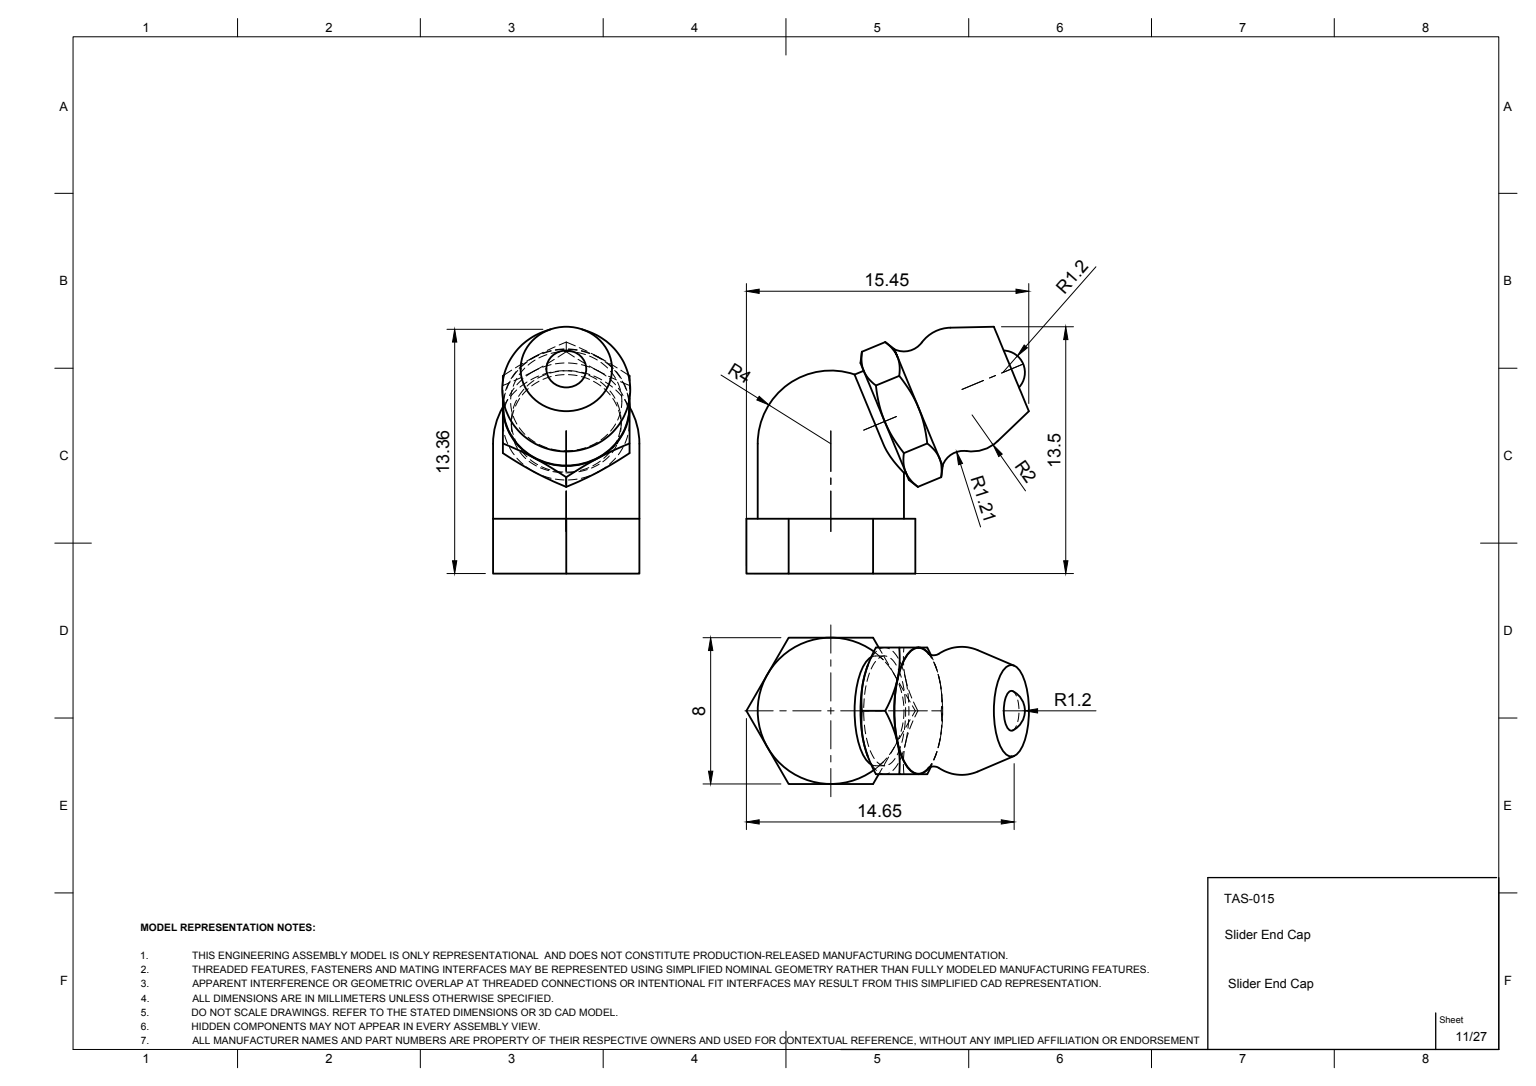
ISO-10303-21;
HEADER;
/* Generated by software containing ST-Developer
 * from STEP Tools, Inc. (www.steptools.com) 
 */

FILE_DESCRIPTION(
/* description */ ('STEP AP214'),
/* implementation_level */ '2;1');

FILE_NAME(
/* name */ 'Slider End Cap.step',
/* time_stamp */ '2026-11-15T14:49:54-08:00',
/* author */ (''),
/* organization */ (''),
/* preprocessor_version */ 'ST-DEVELOPER v20.2',
/* originating_system */ 'Autodesk Translation Framework v15.17.0.0',
/* authorisation */ '');

FILE_SCHEMA (('AUTOMOTIVE_DESIGN { 1 0 10303 214 3 1 1 }'));
ENDSEC;

DATA;
#10=MECHANICAL_DESIGN_GEOMETRIC_PRESENTATION_REPRESENTATION('',(#1106),#66721);
#35=SPHERICAL_SURFACE('',#27201,1.2);
#36=SPHERICAL_SURFACE('',#27220,4.);
#69=TOROIDAL_SURFACE('',#27193,4.25,1.21);
#83=(
BOUNDED_CURVE()
B_SPLINE_CURVE(2,(#39567,#39568,#39569),.UNSPECIFIED.,.F.,.F.)
B_SPLINE_CURVE_WITH_KNOTS((3,3),(-1.38994780338837,-1.00314154055664),
 .UNSPECIFIED.)
CURVE()
GEOMETRIC_REPRESENTATION_ITEM()
RATIONAL_B_SPLINE_CURVE((1.79495951130746,1.93380011269289,1.93380011269289))
REPRESENTATION_ITEM('')
);
#84=(
BOUNDED_CURVE()
B_SPLINE_CURVE(2,(#39570,#39571,#39572),.UNSPECIFIED.,.F.,.F.)
B_SPLINE_CURVE_WITH_KNOTS((3,3),(-1.00619430729118,-0.618602381117838),
 .UNSPECIFIED.)
CURVE()
GEOMETRIC_REPRESENTATION_ITEM()
RATIONAL_B_SPLINE_CURVE((1.93745653739061,1.93745653739061,1.7983534165231))
REPRESENTATION_ITEM('')
);
#85=(
BOUNDED_CURVE()
B_SPLINE_CURVE(2,(#39578,#39579,#39580),.UNSPECIFIED.,.F.,.F.)
B_SPLINE_CURVE_WITH_KNOTS((3,3),(-1.38994780338837,-1.00314154055664),
 .UNSPECIFIED.)
CURVE()
GEOMETRIC_REPRESENTATION_ITEM()
RATIONAL_B_SPLINE_CURVE((1.79495951130745,1.93380011269288,1.93380011269288))
REPRESENTATION_ITEM('')
);
#86=(
BOUNDED_CURVE()
B_SPLINE_CURVE(2,(#39581,#39582,#39583),.UNSPECIFIED.,.F.,.F.)
B_SPLINE_CURVE_WITH_KNOTS((3,3),(-1.00619430729117,-0.618602381117832),
 .UNSPECIFIED.)
CURVE()
GEOMETRIC_REPRESENTATION_ITEM()
RATIONAL_B_SPLINE_CURVE((1.9374565373906,1.9374565373906,1.79835341652309))
REPRESENTATION_ITEM('')
);
#87=(
BOUNDED_CURVE()
B_SPLINE_CURVE(2,(#39705,#39706,#39707),.UNSPECIFIED.,.F.,.F.)
B_SPLINE_CURVE_WITH_KNOTS((3,3),(-1.14357963809553,-0.720457873954785),
 .UNSPECIFIED.)
CURVE()
GEOMETRIC_REPRESENTATION_ITEM()
RATIONAL_B_SPLINE_CURVE((2.10284386262275,2.10284386262275,1.95186646604709))
REPRESENTATION_ITEM('')
);
#88=(
BOUNDED_CURVE()
B_SPLINE_CURVE(2,(#39708,#39709,#39710),.UNSPECIFIED.,.F.,.F.)
B_SPLINE_CURVE_WITH_KNOTS((3,3),(-1.51402948258723,-1.10175646251728),
 .UNSPECIFIED.)
CURVE()
GEOMETRIC_REPRESENTATION_ITEM()
RATIONAL_B_SPLINE_CURVE((1.90498640166842,2.0523376126434,2.0523376126434))
REPRESENTATION_ITEM('')
);
#89=(
BOUNDED_CURVE()
B_SPLINE_CURVE(2,(#39713,#39714,#39715),.UNSPECIFIED.,.F.,.F.)
B_SPLINE_CURVE_WITH_KNOTS((3,3),(-1.00619430729147,-0.618602381118052),
 .UNSPECIFIED.)
CURVE()
GEOMETRIC_REPRESENTATION_ITEM()
RATIONAL_B_SPLINE_CURVE((1.93745653739095,1.93745653739095,1.79835341652342))
REPRESENTATION_ITEM('')
);
#90=(
BOUNDED_CURVE()
B_SPLINE_CURVE(2,(#39716,#39717,#39718),.UNSPECIFIED.,.F.,.F.)
B_SPLINE_CURVE_WITH_KNOTS((3,3),(-1.59428966155348,-1.16547770853232),
 .UNSPECIFIED.)
CURVE()
GEOMETRIC_REPRESENTATION_ITEM()
RATIONAL_B_SPLINE_CURVE((1.97645710138757,2.12933659022722,2.12933659022723))
REPRESENTATION_ITEM('')
);
#91=(
BOUNDED_CURVE()
B_SPLINE_CURVE(2,(#39721,#39722,#39723),.UNSPECIFIED.,.F.,.F.)
B_SPLINE_CURVE_WITH_KNOTS((3,3),(-1.39378623346489,-1.00619430729147),
 .UNSPECIFIED.)
CURVE()
GEOMETRIC_REPRESENTATION_ITEM()
RATIONAL_B_SPLINE_CURVE((1.79835341652342,1.93745653739095,1.93745653739095))
REPRESENTATION_ITEM('')
);
#92=(
BOUNDED_CURVE()
B_SPLINE_CURVE(2,(#39724,#39725,#39726),.UNSPECIFIED.,.F.,.F.)
B_SPLINE_CURVE_WITH_KNOTS((3,3),(-1.00314154055692,-0.616335277725119),
 .UNSPECIFIED.)
CURVE()
GEOMETRIC_REPRESENTATION_ITEM()
RATIONAL_B_SPLINE_CURVE((1.93380011269323,1.93380011269323,1.79495951130777))
REPRESENTATION_ITEM('')
);
#93=(
BOUNDED_CURVE()
B_SPLINE_CURVE(2,(#39729,#39730,#39731),.UNSPECIFIED.,.F.,.F.)
B_SPLINE_CURVE_WITH_KNOTS((3,3),(-1.38994780338873,-1.00314154055692),
 .UNSPECIFIED.)
CURVE()
GEOMETRIC_REPRESENTATION_ITEM()
RATIONAL_B_SPLINE_CURVE((1.79495951130777,1.93380011269323,1.93380011269323))
REPRESENTATION_ITEM('')
);
#94=(
BOUNDED_CURVE()
B_SPLINE_CURVE(2,(#39732,#39733,#39734),.UNSPECIFIED.,.F.,.F.)
B_SPLINE_CURVE_WITH_KNOTS((3,3),(-1.16547770853232,-0.73666575551116),
 .UNSPECIFIED.)
CURVE()
GEOMETRIC_REPRESENTATION_ITEM()
RATIONAL_B_SPLINE_CURVE((2.12933659022723,2.12933659022723,1.97645710138758))
REPRESENTATION_ITEM('')
);
#95=(
BOUNDED_CURVE()
B_SPLINE_CURVE(2,(#39737,#39738,#39739),.UNSPECIFIED.,.F.,.F.)
B_SPLINE_CURVE_WITH_KNOTS((3,3),(-1.56670140223628,-1.14357963809553),
 .UNSPECIFIED.)
CURVE()
GEOMETRIC_REPRESENTATION_ITEM()
RATIONAL_B_SPLINE_CURVE((1.95186646604709,2.10284386262275,2.10284386262275))
REPRESENTATION_ITEM('')
);
#96=(
BOUNDED_CURVE()
B_SPLINE_CURVE(2,(#39740,#39741,#39742),.UNSPECIFIED.,.F.,.F.)
B_SPLINE_CURVE_WITH_KNOTS((3,3),(-1.09872453323964,-0.687236958819027),
 .UNSPECIFIED.)
CURVE()
GEOMETRIC_REPRESENTATION_ITEM()
RATIONAL_B_SPLINE_CURVE((2.04868118794568,2.04868118794568,1.90159249645282))
REPRESENTATION_ITEM('')
);
#97=(
BOUNDED_CURVE()
B_SPLINE_CURVE(2,(#39745,#39746,#39747),.UNSPECIFIED.,.F.,.F.)
B_SPLINE_CURVE_WITH_KNOTS((3,3),(-1.56670140224009,-1.14357963809856),
 .UNSPECIFIED.)
CURVE()
GEOMETRIC_REPRESENTATION_ITEM()
RATIONAL_B_SPLINE_CURVE((1.9518664660505,2.10284386262641,2.10284386262641))
REPRESENTATION_ITEM('')
);
#98=(
BOUNDED_CURVE()
B_SPLINE_CURVE(2,(#39748,#39749,#39750),.UNSPECIFIED.,.F.,.F.)
B_SPLINE_CURVE_WITH_KNOTS((3,3),(-1.10777980342349,-0.69394596557458),
 .UNSPECIFIED.)
CURVE()
GEOMETRIC_REPRESENTATION_ITEM()
RATIONAL_B_SPLINE_CURVE((2.05960365436383,2.05960365436383,1.91173076506448))
REPRESENTATION_ITEM('')
);
#99=(
BOUNDED_CURVE()
B_SPLINE_CURVE(2,(#39753,#39754,#39755),.UNSPECIFIED.,.F.,.F.)
B_SPLINE_CURVE_WITH_KNOTS((3,3),(-1.40141169651805,-1.01225852375907),
 .UNSPECIFIED.)
CURVE()
GEOMETRIC_REPRESENTATION_ITEM()
RATIONAL_B_SPLINE_CURVE((1.80509777991977,1.94472257911162,1.94472257911162))
REPRESENTATION_ITEM('')
);
#100=(
BOUNDED_CURVE()
B_SPLINE_CURVE(2,(#39756,#39757,#39758),.UNSPECIFIED.,.F.,.F.)
B_SPLINE_CURVE_WITH_KNOTS((3,3),(-1.16547770853319,-0.736665755511809),
 .UNSPECIFIED.)
CURVE()
GEOMETRIC_REPRESENTATION_ITEM()
RATIONAL_B_SPLINE_CURVE((2.12933659022829,2.12933659022829,1.97645710138856))
REPRESENTATION_ITEM('')
);
#101=(
BOUNDED_CURVE()
B_SPLINE_CURVE(2,(#39761,#39762,#39763),.UNSPECIFIED.,.F.,.F.)
B_SPLINE_CURVE_WITH_KNOTS((3,3),(-1.40141169651807,-1.01225852375909),
 .UNSPECIFIED.)
CURVE()
GEOMETRIC_REPRESENTATION_ITEM()
RATIONAL_B_SPLINE_CURVE((1.80509777991979,1.94472257911164,1.94472257911164))
REPRESENTATION_ITEM('')
);
#102=(
BOUNDED_CURVE()
B_SPLINE_CURVE(2,(#39764,#39765,#39766),.UNSPECIFIED.,.F.,.F.)
B_SPLINE_CURVE_WITH_KNOTS((3,3),(-1.01225852375907,-0.623105351000092),
 .UNSPECIFIED.)
CURVE()
GEOMETRIC_REPRESENTATION_ITEM()
RATIONAL_B_SPLINE_CURVE((1.94472257911162,1.94472257911162,1.80509777991977))
REPRESENTATION_ITEM('')
);
#103=(
BOUNDED_CURVE()
B_SPLINE_CURVE(2,(#39769,#39770,#39771),.UNSPECIFIED.,.F.,.F.)
B_SPLINE_CURVE_WITH_KNOTS((3,3),(-1.59428966155458,-1.16547770853319),
 .UNSPECIFIED.)
CURVE()
GEOMETRIC_REPRESENTATION_ITEM()
RATIONAL_B_SPLINE_CURVE((1.97645710138856,2.12933659022828,2.12933659022828))
REPRESENTATION_ITEM('')
);
#104=(
BOUNDED_CURVE()
B_SPLINE_CURVE(2,(#39772,#39773,#39774),.UNSPECIFIED.,.F.,.F.)
B_SPLINE_CURVE_WITH_KNOTS((3,3),(-1.01225852375909,-0.623105351000104),
 .UNSPECIFIED.)
CURVE()
GEOMETRIC_REPRESENTATION_ITEM()
RATIONAL_B_SPLINE_CURVE((1.94472257911164,1.94472257911164,1.80509777991979))
REPRESENTATION_ITEM('')
);
#105=(
BOUNDED_CURVE()
B_SPLINE_CURVE(2,(#39777,#39778,#39779),.UNSPECIFIED.,.F.,.F.)
B_SPLINE_CURVE_WITH_KNOTS((3,3),(-1.52161364127241,-1.1077798034235),
 .UNSPECIFIED.)
CURVE()
GEOMETRIC_REPRESENTATION_ITEM()
RATIONAL_B_SPLINE_CURVE((1.91173076506449,2.05960365436384,2.05960365436384))
REPRESENTATION_ITEM('')
);
#106=(
BOUNDED_CURVE()
B_SPLINE_CURVE(2,(#39780,#39781,#39782),.UNSPECIFIED.,.F.,.F.)
B_SPLINE_CURVE_WITH_KNOTS((3,3),(-1.14357963809856,-0.720457873957025),
 .UNSPECIFIED.)
CURVE()
GEOMETRIC_REPRESENTATION_ITEM()
RATIONAL_B_SPLINE_CURVE((2.10284386262641,2.10284386262641,1.95186646605049))
REPRESENTATION_ITEM('')
);
#115=B_SPLINE_CURVE_WITH_KNOTS('',3,(#39589,#39590,#39591,#39592,#39593,
#39594,#39595,#39596,#39597,#39598),.UNSPECIFIED.,.F.,.F.,(4,2,2,2,4),(0.112312904835896,
0.113244103065848,0.226488206131697,0.343893756973101,0.461299307814506),
 .UNSPECIFIED.);
#116=B_SPLINE_CURVE_WITH_KNOTS('',3,(#39602,#39603,#39604,#39605,#39606,
#39607,#39608,#39609,#39610,#39611),.UNSPECIFIED.,.F.,.F.,(4,2,2,2,4),(0.461299307814506,
0.57870485865591,0.696110409497315,0.809354512563163,0.810285710793116),
 .UNSPECIFIED.);
#403=(
BOUNDED_SURFACE()
B_SPLINE_SURFACE(2,2,((#39525,#39526,#39527,#39528,#39529,#39530,#39531,
#39532,#39533),(#39534,#39535,#39536,#39537,#39538,#39539,#39540,#39541,
#39542),(#39543,#39544,#39545,#39546,#39547,#39548,#39549,#39550,#39551)),
 .UNSPECIFIED.,.F.,.T.,.F.)
B_SPLINE_SURFACE_WITH_KNOTS((3,3),(3,2,2,2,3),(-0.371257902576148,0.541962924803503),
(-3.14159265358979,-1.5707963267949,0.,1.5707963267949,3.14159265358979),
 .UNSPECIFIED.)
GEOMETRIC_REPRESENTATION_ITEM()
RATIONAL_B_SPLINE_SURFACE(((1.,0.707106781186548,1.,0.707106781186548,1.,
0.707106781186548,1.,0.707106781186548,1.),(0.897552147568833,0.634665210014471,
0.897552147568833,0.634665210014471,0.897552147568833,0.634665210014471,
0.897552147568833,0.634665210014471,0.897552147568833),(1.,0.707106781186548,
1.,0.707106781186548,1.,0.707106781186548,1.,0.707106781186548,1.)))
REPRESENTATION_ITEM('')
SURFACE()
);
#528=CONICAL_SURFACE('',#27199,2.5,0.371257902576146);
#529=CONICAL_SURFACE('',#27203,4.00000000000001,1.04719755119661);
#530=CONICAL_SURFACE('',#27205,3.46410161513776,1.0471975511966);
#531=CONICAL_SURFACE('',#27247,3.46410161513776,1.0471975511966);
#532=CONICAL_SURFACE('',#27248,3.46410161513776,1.0471975511966);
#533=CONICAL_SURFACE('',#27249,3.46410161513776,1.0471975511966);
#534=CONICAL_SURFACE('',#27250,3.46410161513776,1.0471975511966);
#535=CONICAL_SURFACE('',#27251,3.46410161513776,1.0471975511966);
#536=CONICAL_SURFACE('',#27252,4.00000000000001,1.04719755119661);
#537=CONICAL_SURFACE('',#27253,4.00000000000001,1.04719755119661);
#538=CONICAL_SURFACE('',#27254,4.00000000000001,1.04719755119661);
#539=CONICAL_SURFACE('',#27255,4.00000000000001,1.04719755119661);
#540=CONICAL_SURFACE('',#27256,4.00000000000001,1.04719755119661);
#1044=SHAPE_REPRESENTATION_RELATIONSHIP('SRR','None',#66902,#1075);
#1075=ADVANCED_BREP_SHAPE_REPRESENTATION('',(#1141),#66693);
#1106=STYLED_ITEM('',(#67095),#1141);
#1141=MANIFOLD_SOLID_BREP('Body1',#25672);
#1299=FACE_BOUND('',#4423,.T.);
#1300=FACE_BOUND('',#4425,.T.);
#1301=FACE_BOUND('',#4456,.T.);
#1848=PLANE('',#27222);
#1849=PLANE('',#27228);
#1850=PLANE('',#27234);
#1851=PLANE('',#27235);
#1852=PLANE('',#27236);
#1853=PLANE('',#27237);
#1854=PLANE('',#27238);
#1855=PLANE('',#27239);
#1856=PLANE('',#27240);
#1857=PLANE('',#27241);
#1858=PLANE('',#27242);
#1859=PLANE('',#27243);
#1860=PLANE('',#27244);
#1861=PLANE('',#27245);
#1862=PLANE('',#27246);
#1863=PLANE('',#27257);
#1864=PLANE('',#27258);
#1865=PLANE('',#27259);
#1866=PLANE('',#27260);
#1867=PLANE('',#27261);
#1868=PLANE('',#27262);
#1869=PLANE('',#27263);
#2840=FACE_OUTER_BOUND('',#4413,.T.);
#2841=FACE_OUTER_BOUND('',#4414,.T.);
#2842=FACE_OUTER_BOUND('',#4415,.T.);
#2843=FACE_OUTER_BOUND('',#4416,.T.);
#2844=FACE_OUTER_BOUND('',#4417,.T.);
#2845=FACE_OUTER_BOUND('',#4418,.T.);
#2846=FACE_OUTER_BOUND('',#4419,.T.);
#2847=FACE_OUTER_BOUND('',#4420,.T.);
#2848=FACE_OUTER_BOUND('',#4421,.T.);
#2849=FACE_OUTER_BOUND('',#4422,.T.);
#2850=FACE_OUTER_BOUND('',#4424,.T.);
#2851=FACE_OUTER_BOUND('',#4426,.T.);
#2852=FACE_OUTER_BOUND('',#4427,.T.);
#2853=FACE_OUTER_BOUND('',#4428,.T.);
#2854=FACE_OUTER_BOUND('',#4429,.T.);
#2855=FACE_OUTER_BOUND('',#4430,.T.);
#2856=FACE_OUTER_BOUND('',#4431,.T.);
#2857=FACE_OUTER_BOUND('',#4432,.T.);
#2858=FACE_OUTER_BOUND('',#4433,.T.);
#2859=FACE_OUTER_BOUND('',#4434,.T.);
#2860=FACE_OUTER_BOUND('',#4435,.T.);
#2861=FACE_OUTER_BOUND('',#4436,.T.);
#2862=FACE_OUTER_BOUND('',#4437,.T.);
#2863=FACE_OUTER_BOUND('',#4438,.T.);
#2864=FACE_OUTER_BOUND('',#4439,.T.);
#2865=FACE_OUTER_BOUND('',#4440,.T.);
#2866=FACE_OUTER_BOUND('',#4441,.T.);
#2867=FACE_OUTER_BOUND('',#4442,.T.);
#2868=FACE_OUTER_BOUND('',#4443,.T.);
#2869=FACE_OUTER_BOUND('',#4444,.T.);
#2870=FACE_OUTER_BOUND('',#4445,.T.);
#2871=FACE_OUTER_BOUND('',#4446,.T.);
#2872=FACE_OUTER_BOUND('',#4447,.T.);
#2873=FACE_OUTER_BOUND('',#4448,.T.);
#2874=FACE_OUTER_BOUND('',#4449,.T.);
#2875=FACE_OUTER_BOUND('',#4450,.T.);
#2876=FACE_OUTER_BOUND('',#4451,.T.);
#2877=FACE_OUTER_BOUND('',#4452,.T.);
#2878=FACE_OUTER_BOUND('',#4453,.T.);
#2879=FACE_OUTER_BOUND('',#4454,.T.);
#2880=FACE_OUTER_BOUND('',#4455,.T.);
#4413=EDGE_LOOP('',(#19808,#19809,#19810,#19811));
#4414=EDGE_LOOP('',(#19812,#19813,#19814,#19815));
#4415=EDGE_LOOP('',(#19816,#19817,#19818,#19819));
#4416=EDGE_LOOP('',(#19820));
#4417=EDGE_LOOP('',(#19821,#19822,#19823));
#4418=EDGE_LOOP('',(#19824,#19825,#19826));
#4419=EDGE_LOOP('',(#19827,#19828,#19829,#19830,#19831,#19832));
#4420=EDGE_LOOP('',(#19833,#19834,#19835,#19836,#19837,#19838,#19839,#19840,
#19841,#19842,#19843,#19844,#19845));
#4421=EDGE_LOOP('',(#19846,#19847,#19848,#19849,#19850,#19851));
#4422=EDGE_LOOP('',(#19852,#19853,#19854,#19855,#19856,#19857));
#4423=EDGE_LOOP('',(#19858));
#4424=EDGE_LOOP('',(#19859,#19860,#19861,#19862,#19863,#19864));
#4425=EDGE_LOOP('',(#19865));
#4426=EDGE_LOOP('',(#19866,#19867,#19868));
#4427=EDGE_LOOP('',(#19869,#19870,#19871));
#4428=EDGE_LOOP('',(#19872,#19873,#19874));
#4429=EDGE_LOOP('',(#19875,#19876,#19877));
#4430=EDGE_LOOP('',(#19878,#19879,#19880));
#4431=EDGE_LOOP('',(#19881,#19882,#19883));
#4432=EDGE_LOOP('',(#19884,#19885,#19886,#19887,#19888));
#4433=EDGE_LOOP('',(#19889,#19890,#19891,#19892,#19893));
#4434=EDGE_LOOP('',(#19894,#19895,#19896,#19897,#19898));
#4435=EDGE_LOOP('',(#19899,#19900,#19901,#19902,#19903));
#4436=EDGE_LOOP('',(#19904,#19905,#19906,#19907,#19908));
#4437=EDGE_LOOP('',(#19909,#19910,#19911,#19912,#19913));
#4438=EDGE_LOOP('',(#19914,#19915,#19916,#19917,#19918,#19919));
#4439=EDGE_LOOP('',(#19920,#19921,#19922));
#4440=EDGE_LOOP('',(#19923,#19924,#19925));
#4441=EDGE_LOOP('',(#19926,#19927,#19928));
#4442=EDGE_LOOP('',(#19929,#19930,#19931));
#4443=EDGE_LOOP('',(#19932,#19933,#19934));
#4444=EDGE_LOOP('',(#19935,#19936,#19937));
#4445=EDGE_LOOP('',(#19938,#19939,#19940));
#4446=EDGE_LOOP('',(#19941,#19942,#19943));
#4447=EDGE_LOOP('',(#19944,#19945,#19946));
#4448=EDGE_LOOP('',(#19947,#19948,#19949));
#4449=EDGE_LOOP('',(#19950,#19951,#19952,#19953,#19954,#19955));
#4450=EDGE_LOOP('',(#19956,#19957,#19958,#19959,#19960,#19961));
#4451=EDGE_LOOP('',(#19962,#19963,#19964,#19965,#19966,#19967));
#4452=EDGE_LOOP('',(#19968,#19969,#19970,#19971,#19972,#19973));
#4453=EDGE_LOOP('',(#19974,#19975,#19976,#19977,#19978,#19979));
#4454=EDGE_LOOP('',(#19980,#19981,#19982,#19983,#19984,#19985));
#4455=EDGE_LOOP('',(#19986));
#4456=EDGE_LOOP('',(#19987));
#6516=LINE('',#39557,#8505);
#6517=LINE('',#39600,#8506);
#6518=LINE('',#39619,#8507);
#6519=LINE('',#39656,#8508);
#6520=LINE('',#39657,#8509);
#6521=LINE('',#39660,#8510);
#6522=LINE('',#39661,#8511);
#6523=LINE('',#39664,#8512);
#6524=LINE('',#39665,#8513);
#6525=LINE('',#39668,#8514);
#6526=LINE('',#39669,#8515);
#6527=LINE('',#39672,#8516);
#6528=LINE('',#39673,#8517);
#6529=LINE('',#39676,#8518);
#6530=LINE('',#39677,#8519);
#6531=LINE('',#39681,#8520);
#6532=LINE('',#39682,#8521);
#6533=LINE('',#39683,#8522);
#6534=LINE('',#39686,#8523);
#6535=LINE('',#39687,#8524);
#6536=LINE('',#39690,#8525);
#6537=LINE('',#39691,#8526);
#6538=LINE('',#39694,#8527);
#6539=LINE('',#39695,#8528);
#6540=LINE('',#39698,#8529);
#6541=LINE('',#39699,#8530);
#6542=LINE('',#39701,#8531);
#6543=LINE('',#39784,#8532);
#6544=LINE('',#39785,#8533);
#6545=LINE('',#39787,#8534);
#6546=LINE('',#39789,#8535);
#6547=LINE('',#39791,#8536);
#6548=LINE('',#39793,#8537);
#8505=VECTOR('',#32107,2.5);
#8506=VECTOR('',#32126,3.);
#8507=VECTOR('',#32137,4.);
#8508=VECTOR('',#32180,1000.);
#8509=VECTOR('',#32181,1000.);
#8510=VECTOR('',#32184,1000.);
#8511=VECTOR('',#32185,1000.);
#8512=VECTOR('',#32188,1000.);
#8513=VECTOR('',#32189,1000.);
#8514=VECTOR('',#32192,1000.);
#8515=VECTOR('',#32193,1000.);
#8516=VECTOR('',#32196,1000.);
#8517=VECTOR('',#32197,1000.);
#8518=VECTOR('',#32200,1000.);
#8519=VECTOR('',#32201,1000.);
#8520=VECTOR('',#32204,1000.);
#8521=VECTOR('',#32205,1000.);
#8522=VECTOR('',#32206,1000.);
#8523=VECTOR('',#32209,1000.);
#8524=VECTOR('',#32210,1000.);
#8525=VECTOR('',#32213,1000.);
#8526=VECTOR('',#32214,1000.);
#8527=VECTOR('',#32217,1000.);
#8528=VECTOR('',#32218,1000.);
#8529=VECTOR('',#32221,1000.);
#8530=VECTOR('',#32222,1000.);
#8531=VECTOR('',#32225,1000.);
#8532=VECTOR('',#32250,1000.);
#8533=VECTOR('',#32251,1000.);
#8534=VECTOR('',#32254,1000.);
#8535=VECTOR('',#32257,1000.);
#8536=VECTOR('',#32260,1000.);
#8537=VECTOR('',#32263,1000.);
#9952=CIRCLE('',#27194,3.44123551017618);
#9953=CIRCLE('',#27195,1.21);
#9954=CIRCLE('',#27196,3.21339563862929);
#9955=CIRCLE('',#27197,2.);
#9956=CIRCLE('',#27198,3.36374346224613);
#9957=CIRCLE('',#27200,2.5);
#9958=CIRCLE('',#27202,1.09087121146357);
#9959=CIRCLE('',#27204,3.46410161513777);
#9960=CIRCLE('',#27206,3.46410161513775);
#9961=CIRCLE('',#27208,3.);
#9962=CIRCLE('',#27209,3.);
#9963=CIRCLE('',#27211,4.);
#9964=CIRCLE('',#27212,4.);
#9965=CIRCLE('',#27213,4.);
#9966=CIRCLE('',#27214,4.);
#9967=CIRCLE('',#27215,4.);
#9968=CIRCLE('',#27216,4.);
#9969=CIRCLE('',#27217,4.);
#9970=CIRCLE('',#27218,4.);
#9971=CIRCLE('',#27219,4.);
#9972=CIRCLE('',#27221,4.);
#9973=CIRCLE('',#27223,3.46410161513776);
#9974=CIRCLE('',#27224,3.46410161513777);
#9975=CIRCLE('',#27225,3.46410161513777);
#9976=CIRCLE('',#27226,3.46410161513777);
#9977=CIRCLE('',#27227,3.46410161513777);
#9978=CIRCLE('',#27229,3.46410161513775);
#9979=CIRCLE('',#27230,3.46410161513775);
#9980=CIRCLE('',#27231,3.46410161513775);
#9981=CIRCLE('',#27232,3.46410161513775);
#9982=CIRCLE('',#27233,3.46410161513776);
#11707=VERTEX_POINT('',#39520);
#11708=VERTEX_POINT('',#39522);
#11709=VERTEX_POINT('',#39552);
#11710=VERTEX_POINT('',#39556);
#11711=VERTEX_POINT('',#39560);
#11712=VERTEX_POINT('',#39563);
#11713=VERTEX_POINT('',#39564);
#11714=VERTEX_POINT('',#39566);
#11715=VERTEX_POINT('',#39574);
#11716=VERTEX_POINT('',#39575);
#11717=VERTEX_POINT('',#39577);
#11718=VERTEX_POINT('',#39585);
#11719=VERTEX_POINT('',#39586);
#11720=VERTEX_POINT('',#39588);
#11721=VERTEX_POINT('',#39599);
#11722=VERTEX_POINT('',#39613);
#11723=VERTEX_POINT('',#39615);
#11724=VERTEX_POINT('',#39618);
#11725=VERTEX_POINT('',#39620);
#11726=VERTEX_POINT('',#39622);
#11727=VERTEX_POINT('',#39624);
#11728=VERTEX_POINT('',#39626);
#11729=VERTEX_POINT('',#39628);
#11730=VERTEX_POINT('',#39632);
#11731=VERTEX_POINT('',#39635);
#11732=VERTEX_POINT('',#39637);
#11733=VERTEX_POINT('',#39639);
#11734=VERTEX_POINT('',#39641);
#11735=VERTEX_POINT('',#39645);
#11736=VERTEX_POINT('',#39647);
#11737=VERTEX_POINT('',#39649);
#11738=VERTEX_POINT('',#39651);
#11739=VERTEX_POINT('',#39655);
#11740=VERTEX_POINT('',#39659);
#11741=VERTEX_POINT('',#39663);
#11742=VERTEX_POINT('',#39667);
#11743=VERTEX_POINT('',#39671);
#11744=VERTEX_POINT('',#39675);
#11745=VERTEX_POINT('',#39679);
#11746=VERTEX_POINT('',#39680);
#11747=VERTEX_POINT('',#39685);
#11748=VERTEX_POINT('',#39689);
#11749=VERTEX_POINT('',#39693);
#11750=VERTEX_POINT('',#39697);
#11751=VERTEX_POINT('',#39704);
#11752=VERTEX_POINT('',#39712);
#11753=VERTEX_POINT('',#39720);
#11754=VERTEX_POINT('',#39728);
#11755=VERTEX_POINT('',#39736);
#11756=VERTEX_POINT('',#39744);
#11757=VERTEX_POINT('',#39752);
#11758=VERTEX_POINT('',#39760);
#11759=VERTEX_POINT('',#39768);
#11760=VERTEX_POINT('',#39776);
#14597=EDGE_CURVE('',#11707,#11707,#9952,.T.);
#14598=EDGE_CURVE('',#11707,#11708,#9953,.T.);
#14599=EDGE_CURVE('',#11708,#11708,#9954,.T.);
#14600=EDGE_CURVE('',#11708,#11709,#9955,.T.);
#14601=EDGE_CURVE('',#11709,#11709,#9956,.T.);
#14602=EDGE_CURVE('',#11709,#11710,#6516,.T.);
#14603=EDGE_CURVE('',#11710,#11710,#9957,.T.);
#14604=EDGE_CURVE('',#11711,#11711,#9958,.T.);
#14605=EDGE_CURVE('',#11712,#11713,#9959,.T.);
#14606=EDGE_CURVE('',#11714,#11713,#83,.T.);
#14607=EDGE_CURVE('',#11712,#11714,#84,.T.);
#14608=EDGE_CURVE('',#11715,#11716,#9960,.T.);
#14609=EDGE_CURVE('',#11717,#11716,#85,.T.);
#14610=EDGE_CURVE('',#11715,#11717,#86,.T.);
#14611=EDGE_CURVE('',#11718,#11719,#9961,.T.);
#14612=EDGE_CURVE('',#11720,#11718,#115,.F.);
#14613=EDGE_CURVE('',#11720,#11721,#6517,.T.);
#14614=EDGE_CURVE('',#11721,#11721,#9962,.T.);
#14615=EDGE_CURVE('',#11719,#11720,#116,.F.);
#14616=EDGE_CURVE('',#11719,#11722,#9963,.T.);
#14617=EDGE_CURVE('',#11723,#11718,#9964,.T.);
#14618=EDGE_CURVE('',#11722,#11723,#9965,.T.);
#14619=EDGE_CURVE('',#11722,#11724,#6518,.T.);
#14620=EDGE_CURVE('',#11724,#11725,#9966,.T.);
#14621=EDGE_CURVE('',#11725,#11726,#9967,.T.);
#14622=EDGE_CURVE('',#11726,#11727,#9968,.T.);
#14623=EDGE_CURVE('',#11727,#11728,#9969,.T.);
#14624=EDGE_CURVE('',#11728,#11729,#9970,.T.);
#14625=EDGE_CURVE('',#11729,#11724,#9971,.T.);
#14626=EDGE_CURVE('',#11723,#11730,#9972,.T.);
#14627=EDGE_CURVE('',#11713,#11731,#9973,.T.);
#14628=EDGE_CURVE('',#11732,#11712,#9974,.T.);
#14629=EDGE_CURVE('',#11733,#11732,#9975,.T.);
#14630=EDGE_CURVE('',#11734,#11733,#9976,.T.);
#14631=EDGE_CURVE('',#11731,#11734,#9977,.T.);
#14632=EDGE_CURVE('',#11716,#11735,#9978,.T.);
#14633=EDGE_CURVE('',#11736,#11715,#9979,.T.);
#14634=EDGE_CURVE('',#11737,#11736,#9980,.T.);
#14635=EDGE_CURVE('',#11738,#11737,#9981,.T.);
#14636=EDGE_CURVE('',#11738,#11735,#9982,.T.);
#14637=EDGE_CURVE('',#11739,#11727,#6519,.T.);
#14638=EDGE_CURVE('',#11728,#11739,#6520,.T.);
#14639=EDGE_CURVE('',#11740,#11728,#6521,.T.);
#14640=EDGE_CURVE('',#11729,#11740,#6522,.T.);
#14641=EDGE_CURVE('',#11741,#11729,#6523,.T.);
#14642=EDGE_CURVE('',#11724,#11741,#6524,.T.);
#14643=EDGE_CURVE('',#11742,#11724,#6525,.T.);
#14644=EDGE_CURVE('',#11725,#11742,#6526,.T.);
#14645=EDGE_CURVE('',#11743,#11725,#6527,.T.);
#14646=EDGE_CURVE('',#11726,#11743,#6528,.T.);
#14647=EDGE_CURVE('',#11744,#11726,#6529,.T.);
#14648=EDGE_CURVE('',#11727,#11744,#6530,.T.);
#14649=EDGE_CURVE('',#11745,#11746,#6531,.T.);
#14650=EDGE_CURVE('',#11741,#11745,#6532,.T.);
#14651=EDGE_CURVE('',#11740,#11746,#6533,.T.);
#14652=EDGE_CURVE('',#11747,#11745,#6534,.T.);
#14653=EDGE_CURVE('',#11742,#11747,#6535,.T.);
#14654=EDGE_CURVE('',#11748,#11747,#6536,.T.);
#14655=EDGE_CURVE('',#11743,#11748,#6537,.T.);
#14656=EDGE_CURVE('',#11749,#11748,#6538,.T.);
#14657=EDGE_CURVE('',#11744,#11749,#6539,.T.);
#14658=EDGE_CURVE('',#11750,#11749,#6540,.T.);
#14659=EDGE_CURVE('',#11739,#11750,#6541,.T.);
#14660=EDGE_CURVE('',#11746,#11750,#6542,.T.);
#14661=EDGE_CURVE('',#11736,#11751,#87,.T.);
#14662=EDGE_CURVE('',#11751,#11715,#88,.T.);
#14663=EDGE_CURVE('',#11737,#11752,#89,.T.);
#14664=EDGE_CURVE('',#11752,#11736,#90,.T.);
#14665=EDGE_CURVE('',#11753,#11737,#91,.T.);
#14666=EDGE_CURVE('',#11738,#11753,#92,.T.);
#14667=EDGE_CURVE('',#11754,#11738,#93,.T.);
#14668=EDGE_CURVE('',#11735,#11754,#94,.T.);
#14669=EDGE_CURVE('',#11755,#11735,#95,.T.);
#14670=EDGE_CURVE('',#11716,#11755,#96,.T.);
#14671=EDGE_CURVE('',#11756,#11731,#97,.T.);
#14672=EDGE_CURVE('',#11713,#11756,#98,.T.);
#14673=EDGE_CURVE('',#11757,#11734,#99,.T.);
#14674=EDGE_CURVE('',#11731,#11757,#100,.T.);
#14675=EDGE_CURVE('',#11758,#11733,#101,.T.);
#14676=EDGE_CURVE('',#11734,#11758,#102,.T.);
#14677=EDGE_CURVE('',#11759,#11732,#103,.T.);
#14678=EDGE_CURVE('',#11733,#11759,#104,.T.);
#14679=EDGE_CURVE('',#11760,#11712,#105,.T.);
#14680=EDGE_CURVE('',#11732,#11760,#106,.T.);
#14681=EDGE_CURVE('',#11753,#11714,#6543,.T.);
#14682=EDGE_CURVE('',#11752,#11760,#6544,.T.);
#14683=EDGE_CURVE('',#11751,#11759,#6545,.T.);
#14684=EDGE_CURVE('',#11717,#11758,#6546,.T.);
#14685=EDGE_CURVE('',#11755,#11757,#6547,.T.);
#14686=EDGE_CURVE('',#11754,#11756,#6548,.T.);
#19808=ORIENTED_EDGE('',*,*,#14597,.T.);
#19809=ORIENTED_EDGE('',*,*,#14598,.T.);
#19810=ORIENTED_EDGE('',*,*,#14599,.T.);
#19811=ORIENTED_EDGE('',*,*,#14598,.F.);
#19812=ORIENTED_EDGE('',*,*,#14599,.F.);
#19813=ORIENTED_EDGE('',*,*,#14600,.T.);
#19814=ORIENTED_EDGE('',*,*,#14601,.T.);
#19815=ORIENTED_EDGE('',*,*,#14600,.F.);
#19816=ORIENTED_EDGE('',*,*,#14601,.F.);
#19817=ORIENTED_EDGE('',*,*,#14602,.T.);
#19818=ORIENTED_EDGE('',*,*,#14603,.T.);
#19819=ORIENTED_EDGE('',*,*,#14602,.F.);
#19820=ORIENTED_EDGE('',*,*,#14604,.F.);
#19821=ORIENTED_EDGE('',*,*,#14605,.T.);
#19822=ORIENTED_EDGE('',*,*,#14606,.F.);
#19823=ORIENTED_EDGE('',*,*,#14607,.F.);
#19824=ORIENTED_EDGE('',*,*,#14608,.T.);
#19825=ORIENTED_EDGE('',*,*,#14609,.F.);
#19826=ORIENTED_EDGE('',*,*,#14610,.F.);
#19827=ORIENTED_EDGE('',*,*,#14611,.F.);
#19828=ORIENTED_EDGE('',*,*,#14612,.F.);
#19829=ORIENTED_EDGE('',*,*,#14613,.T.);
#19830=ORIENTED_EDGE('',*,*,#14614,.T.);
#19831=ORIENTED_EDGE('',*,*,#14613,.F.);
#19832=ORIENTED_EDGE('',*,*,#14615,.F.);
#19833=ORIENTED_EDGE('',*,*,#14616,.F.);
#19834=ORIENTED_EDGE('',*,*,#14615,.T.);
#19835=ORIENTED_EDGE('',*,*,#14612,.T.);
#19836=ORIENTED_EDGE('',*,*,#14617,.F.);
#19837=ORIENTED_EDGE('',*,*,#14618,.F.);
#19838=ORIENTED_EDGE('',*,*,#14619,.T.);
#19839=ORIENTED_EDGE('',*,*,#14620,.T.);
#19840=ORIENTED_EDGE('',*,*,#14621,.T.);
#19841=ORIENTED_EDGE('',*,*,#14622,.T.);
#19842=ORIENTED_EDGE('',*,*,#14623,.T.);
#19843=ORIENTED_EDGE('',*,*,#14624,.T.);
#19844=ORIENTED_EDGE('',*,*,#14625,.T.);
#19845=ORIENTED_EDGE('',*,*,#14619,.F.);
#19846=ORIENTED_EDGE('',*,*,#14616,.T.);
#19847=ORIENTED_EDGE('',*,*,#14618,.T.);
#19848=ORIENTED_EDGE('',*,*,#14626,.T.);
#19849=ORIENTED_EDGE('',*,*,#14626,.F.);
#19850=ORIENTED_EDGE('',*,*,#14617,.T.);
#19851=ORIENTED_EDGE('',*,*,#14611,.T.);
#19852=ORIENTED_EDGE('',*,*,#14627,.F.);
#19853=ORIENTED_EDGE('',*,*,#14605,.F.);
#19854=ORIENTED_EDGE('',*,*,#14628,.F.);
#19855=ORIENTED_EDGE('',*,*,#14629,.F.);
#19856=ORIENTED_EDGE('',*,*,#14630,.F.);
#19857=ORIENTED_EDGE('',*,*,#14631,.F.);
#19858=ORIENTED_EDGE('',*,*,#14597,.F.);
#19859=ORIENTED_EDGE('',*,*,#14632,.F.);
#19860=ORIENTED_EDGE('',*,*,#14608,.F.);
#19861=ORIENTED_EDGE('',*,*,#14633,.F.);
#19862=ORIENTED_EDGE('',*,*,#14634,.F.);
#19863=ORIENTED_EDGE('',*,*,#14635,.F.);
#19864=ORIENTED_EDGE('',*,*,#14636,.T.);
#19865=ORIENTED_EDGE('',*,*,#14614,.F.);
#19866=ORIENTED_EDGE('',*,*,#14623,.F.);
#19867=ORIENTED_EDGE('',*,*,#14637,.F.);
#19868=ORIENTED_EDGE('',*,*,#14638,.F.);
#19869=ORIENTED_EDGE('',*,*,#14624,.F.);
#19870=ORIENTED_EDGE('',*,*,#14639,.F.);
#19871=ORIENTED_EDGE('',*,*,#14640,.F.);
#19872=ORIENTED_EDGE('',*,*,#14625,.F.);
#19873=ORIENTED_EDGE('',*,*,#14641,.F.);
#19874=ORIENTED_EDGE('',*,*,#14642,.F.);
#19875=ORIENTED_EDGE('',*,*,#14620,.F.);
#19876=ORIENTED_EDGE('',*,*,#14643,.F.);
#19877=ORIENTED_EDGE('',*,*,#14644,.F.);
#19878=ORIENTED_EDGE('',*,*,#14621,.F.);
#19879=ORIENTED_EDGE('',*,*,#14645,.F.);
#19880=ORIENTED_EDGE('',*,*,#14646,.F.);
#19881=ORIENTED_EDGE('',*,*,#14622,.F.);
#19882=ORIENTED_EDGE('',*,*,#14647,.F.);
#19883=ORIENTED_EDGE('',*,*,#14648,.F.);
#19884=ORIENTED_EDGE('',*,*,#14649,.F.);
#19885=ORIENTED_EDGE('',*,*,#14650,.F.);
#19886=ORIENTED_EDGE('',*,*,#14641,.T.);
#19887=ORIENTED_EDGE('',*,*,#14640,.T.);
#19888=ORIENTED_EDGE('',*,*,#14651,.T.);
#19889=ORIENTED_EDGE('',*,*,#14652,.F.);
#19890=ORIENTED_EDGE('',*,*,#14653,.F.);
#19891=ORIENTED_EDGE('',*,*,#14643,.T.);
#19892=ORIENTED_EDGE('',*,*,#14642,.T.);
#19893=ORIENTED_EDGE('',*,*,#14650,.T.);
#19894=ORIENTED_EDGE('',*,*,#14654,.F.);
#19895=ORIENTED_EDGE('',*,*,#14655,.F.);
#19896=ORIENTED_EDGE('',*,*,#14645,.T.);
#19897=ORIENTED_EDGE('',*,*,#14644,.T.);
#19898=ORIENTED_EDGE('',*,*,#14653,.T.);
#19899=ORIENTED_EDGE('',*,*,#14656,.F.);
#19900=ORIENTED_EDGE('',*,*,#14657,.F.);
#19901=ORIENTED_EDGE('',*,*,#14647,.T.);
#19902=ORIENTED_EDGE('',*,*,#14646,.T.);
#19903=ORIENTED_EDGE('',*,*,#14655,.T.);
#19904=ORIENTED_EDGE('',*,*,#14658,.F.);
#19905=ORIENTED_EDGE('',*,*,#14659,.F.);
#19906=ORIENTED_EDGE('',*,*,#14637,.T.);
#19907=ORIENTED_EDGE('',*,*,#14648,.T.);
#19908=ORIENTED_EDGE('',*,*,#14657,.T.);
#19909=ORIENTED_EDGE('',*,*,#14660,.F.);
#19910=ORIENTED_EDGE('',*,*,#14651,.F.);
#19911=ORIENTED_EDGE('',*,*,#14639,.T.);
#19912=ORIENTED_EDGE('',*,*,#14638,.T.);
#19913=ORIENTED_EDGE('',*,*,#14659,.T.);
#19914=ORIENTED_EDGE('',*,*,#14649,.T.);
#19915=ORIENTED_EDGE('',*,*,#14660,.T.);
#19916=ORIENTED_EDGE('',*,*,#14658,.T.);
#19917=ORIENTED_EDGE('',*,*,#14656,.T.);
#19918=ORIENTED_EDGE('',*,*,#14654,.T.);
#19919=ORIENTED_EDGE('',*,*,#14652,.T.);
#19920=ORIENTED_EDGE('',*,*,#14661,.F.);
#19921=ORIENTED_EDGE('',*,*,#14633,.T.);
#19922=ORIENTED_EDGE('',*,*,#14662,.F.);
#19923=ORIENTED_EDGE('',*,*,#14663,.F.);
#19924=ORIENTED_EDGE('',*,*,#14634,.T.);
#19925=ORIENTED_EDGE('',*,*,#14664,.F.);
#19926=ORIENTED_EDGE('',*,*,#14635,.T.);
#19927=ORIENTED_EDGE('',*,*,#14665,.F.);
#19928=ORIENTED_EDGE('',*,*,#14666,.F.);
#19929=ORIENTED_EDGE('',*,*,#14636,.F.);
#19930=ORIENTED_EDGE('',*,*,#14667,.F.);
#19931=ORIENTED_EDGE('',*,*,#14668,.F.);
#19932=ORIENTED_EDGE('',*,*,#14632,.T.);
#19933=ORIENTED_EDGE('',*,*,#14669,.F.);
#19934=ORIENTED_EDGE('',*,*,#14670,.F.);
#19935=ORIENTED_EDGE('',*,*,#14627,.T.);
#19936=ORIENTED_EDGE('',*,*,#14671,.F.);
#19937=ORIENTED_EDGE('',*,*,#14672,.F.);
#19938=ORIENTED_EDGE('',*,*,#14631,.T.);
#19939=ORIENTED_EDGE('',*,*,#14673,.F.);
#19940=ORIENTED_EDGE('',*,*,#14674,.F.);
#19941=ORIENTED_EDGE('',*,*,#14630,.T.);
#19942=ORIENTED_EDGE('',*,*,#14675,.F.);
#19943=ORIENTED_EDGE('',*,*,#14676,.F.);
#19944=ORIENTED_EDGE('',*,*,#14629,.T.);
#19945=ORIENTED_EDGE('',*,*,#14677,.F.);
#19946=ORIENTED_EDGE('',*,*,#14678,.F.);
#19947=ORIENTED_EDGE('',*,*,#14628,.T.);
#19948=ORIENTED_EDGE('',*,*,#14679,.F.);
#19949=ORIENTED_EDGE('',*,*,#14680,.F.);
#19950=ORIENTED_EDGE('',*,*,#14681,.F.);
#19951=ORIENTED_EDGE('',*,*,#14665,.T.);
#19952=ORIENTED_EDGE('',*,*,#14663,.T.);
#19953=ORIENTED_EDGE('',*,*,#14682,.T.);
#19954=ORIENTED_EDGE('',*,*,#14679,.T.);
#19955=ORIENTED_EDGE('',*,*,#14607,.T.);
#19956=ORIENTED_EDGE('',*,*,#14682,.F.);
#19957=ORIENTED_EDGE('',*,*,#14664,.T.);
#19958=ORIENTED_EDGE('',*,*,#14661,.T.);
#19959=ORIENTED_EDGE('',*,*,#14683,.T.);
#19960=ORIENTED_EDGE('',*,*,#14677,.T.);
#19961=ORIENTED_EDGE('',*,*,#14680,.T.);
#19962=ORIENTED_EDGE('',*,*,#14683,.F.);
#19963=ORIENTED_EDGE('',*,*,#14662,.T.);
#19964=ORIENTED_EDGE('',*,*,#14610,.T.);
#19965=ORIENTED_EDGE('',*,*,#14684,.T.);
#19966=ORIENTED_EDGE('',*,*,#14675,.T.);
#19967=ORIENTED_EDGE('',*,*,#14678,.T.);
#19968=ORIENTED_EDGE('',*,*,#14684,.F.);
#19969=ORIENTED_EDGE('',*,*,#14609,.T.);
#19970=ORIENTED_EDGE('',*,*,#14670,.T.);
#19971=ORIENTED_EDGE('',*,*,#14685,.T.);
#19972=ORIENTED_EDGE('',*,*,#14673,.T.);
#19973=ORIENTED_EDGE('',*,*,#14676,.T.);
#19974=ORIENTED_EDGE('',*,*,#14685,.F.);
#19975=ORIENTED_EDGE('',*,*,#14669,.T.);
#19976=ORIENTED_EDGE('',*,*,#14668,.T.);
#19977=ORIENTED_EDGE('',*,*,#14686,.T.);
#19978=ORIENTED_EDGE('',*,*,#14671,.T.);
#19979=ORIENTED_EDGE('',*,*,#14674,.T.);
#19980=ORIENTED_EDGE('',*,*,#14686,.F.);
#19981=ORIENTED_EDGE('',*,*,#14667,.T.);
#19982=ORIENTED_EDGE('',*,*,#14666,.T.);
#19983=ORIENTED_EDGE('',*,*,#14681,.T.);
#19984=ORIENTED_EDGE('',*,*,#14606,.T.);
#19985=ORIENTED_EDGE('',*,*,#14672,.T.);
#19986=ORIENTED_EDGE('',*,*,#14603,.F.);
#19987=ORIENTED_EDGE('',*,*,#14604,.T.);
#24018=CYLINDRICAL_SURFACE('',#27207,3.);
#24019=CYLINDRICAL_SURFACE('',#27210,4.);
#24793=ADVANCED_FACE('',(#2840),#69,.F.);
#24794=ADVANCED_FACE('',(#2841),#403,.F.);
#24795=ADVANCED_FACE('',(#2842),#528,.T.);
#24796=ADVANCED_FACE('',(#2843),#35,.T.);
#24797=ADVANCED_FACE('',(#2844),#529,.T.);
#24798=ADVANCED_FACE('',(#2845),#530,.T.);
#24799=ADVANCED_FACE('',(#2846),#24018,.T.);
#24800=ADVANCED_FACE('',(#2847),#24019,.T.);
#24801=ADVANCED_FACE('',(#2848),#36,.T.);
#24802=ADVANCED_FACE('',(#2849,#1299),#1848,.F.);
#24803=ADVANCED_FACE('',(#2850,#1300),#1849,.F.);
#24804=ADVANCED_FACE('',(#2851),#1850,.F.);
#24805=ADVANCED_FACE('',(#2852),#1851,.F.);
#24806=ADVANCED_FACE('',(#2853),#1852,.F.);
#24807=ADVANCED_FACE('',(#2854),#1853,.F.);
#24808=ADVANCED_FACE('',(#2855),#1854,.F.);
#24809=ADVANCED_FACE('',(#2856),#1855,.F.);
#24810=ADVANCED_FACE('',(#2857),#1856,.T.);
#24811=ADVANCED_FACE('',(#2858),#1857,.T.);
#24812=ADVANCED_FACE('',(#2859),#1858,.T.);
#24813=ADVANCED_FACE('',(#2860),#1859,.T.);
#24814=ADVANCED_FACE('',(#2861),#1860,.T.);
#24815=ADVANCED_FACE('',(#2862),#1861,.T.);
#24816=ADVANCED_FACE('',(#2863),#1862,.T.);
#24817=ADVANCED_FACE('',(#2864),#531,.T.);
#24818=ADVANCED_FACE('',(#2865),#532,.T.);
#24819=ADVANCED_FACE('',(#2866),#533,.T.);
#24820=ADVANCED_FACE('',(#2867),#534,.T.);
#24821=ADVANCED_FACE('',(#2868),#535,.T.);
#24822=ADVANCED_FACE('',(#2869),#536,.T.);
#24823=ADVANCED_FACE('',(#2870),#537,.T.);
#24824=ADVANCED_FACE('',(#2871),#538,.T.);
#24825=ADVANCED_FACE('',(#2872),#539,.T.);
#24826=ADVANCED_FACE('',(#2873),#540,.T.);
#24827=ADVANCED_FACE('',(#2874),#1863,.T.);
#24828=ADVANCED_FACE('',(#2875),#1864,.T.);
#24829=ADVANCED_FACE('',(#2876),#1865,.T.);
#24830=ADVANCED_FACE('',(#2877),#1866,.T.);
#24831=ADVANCED_FACE('',(#2878),#1867,.T.);
#24832=ADVANCED_FACE('',(#2879),#1868,.T.);
#24833=ADVANCED_FACE('',(#2880,#1301),#1869,.F.);
#25672=CLOSED_SHELL('',(#24793,#24794,#24795,#24796,#24797,#24798,#24799,
#24800,#24801,#24802,#24803,#24804,#24805,#24806,#24807,#24808,#24809,#24810,
#24811,#24812,#24813,#24814,#24815,#24816,#24817,#24818,#24819,#24820,#24821,
#24822,#24823,#24824,#24825,#24826,#24827,#24828,#24829,#24830,#24831,#24832,
#24833));
#27192=AXIS2_PLACEMENT_3D('',#39518,#32091,#32092);
#27193=AXIS2_PLACEMENT_3D('',#39519,#32093,#32094);
#27194=AXIS2_PLACEMENT_3D('',#39521,#32095,#32096);
#27195=AXIS2_PLACEMENT_3D('',#39523,#32097,#32098);
#27196=AXIS2_PLACEMENT_3D('',#39524,#32099,#32100);
#27197=AXIS2_PLACEMENT_3D('',#39553,#32101,#32102);
#27198=AXIS2_PLACEMENT_3D('',#39554,#32103,#32104);
#27199=AXIS2_PLACEMENT_3D('',#39555,#32105,#32106);
#27200=AXIS2_PLACEMENT_3D('',#39558,#32108,#32109);
#27201=AXIS2_PLACEMENT_3D('',#39559,#32110,#32111);
#27202=AXIS2_PLACEMENT_3D('',#39561,#32112,#32113);
#27203=AXIS2_PLACEMENT_3D('',#39562,#32114,#32115);
#27204=AXIS2_PLACEMENT_3D('',#39565,#32116,#32117);
#27205=AXIS2_PLACEMENT_3D('',#39573,#32118,#32119);
#27206=AXIS2_PLACEMENT_3D('',#39576,#32120,#32121);
#27207=AXIS2_PLACEMENT_3D('',#39584,#32122,#32123);
#27208=AXIS2_PLACEMENT_3D('',#39587,#32124,#32125);
#27209=AXIS2_PLACEMENT_3D('',#39601,#32127,#32128);
#27210=AXIS2_PLACEMENT_3D('',#39612,#32129,#32130);
#27211=AXIS2_PLACEMENT_3D('',#39614,#32131,#32132);
#27212=AXIS2_PLACEMENT_3D('',#39616,#32133,#32134);
#27213=AXIS2_PLACEMENT_3D('',#39617,#32135,#32136);
#27214=AXIS2_PLACEMENT_3D('',#39621,#32138,#32139);
#27215=AXIS2_PLACEMENT_3D('',#39623,#32140,#32141);
#27216=AXIS2_PLACEMENT_3D('',#39625,#32142,#32143);
#27217=AXIS2_PLACEMENT_3D('',#39627,#32144,#32145);
#27218=AXIS2_PLACEMENT_3D('',#39629,#32146,#32147);
#27219=AXIS2_PLACEMENT_3D('',#39630,#32148,#32149);
#27220=AXIS2_PLACEMENT_3D('',#39631,#32150,#32151);
#27221=AXIS2_PLACEMENT_3D('',#39633,#32152,#32153);
#27222=AXIS2_PLACEMENT_3D('',#39634,#32154,#32155);
#27223=AXIS2_PLACEMENT_3D('',#39636,#32156,#32157);
#27224=AXIS2_PLACEMENT_3D('',#39638,#32158,#32159);
#27225=AXIS2_PLACEMENT_3D('',#39640,#32160,#32161);
#27226=AXIS2_PLACEMENT_3D('',#39642,#32162,#32163);
#27227=AXIS2_PLACEMENT_3D('',#39643,#32164,#32165);
#27228=AXIS2_PLACEMENT_3D('',#39644,#32166,#32167);
#27229=AXIS2_PLACEMENT_3D('',#39646,#32168,#32169);
#27230=AXIS2_PLACEMENT_3D('',#39648,#32170,#32171);
#27231=AXIS2_PLACEMENT_3D('',#39650,#32172,#32173);
#27232=AXIS2_PLACEMENT_3D('',#39652,#32174,#32175);
#27233=AXIS2_PLACEMENT_3D('',#39653,#32176,#32177);
#27234=AXIS2_PLACEMENT_3D('',#39654,#32178,#32179);
#27235=AXIS2_PLACEMENT_3D('',#39658,#32182,#32183);
#27236=AXIS2_PLACEMENT_3D('',#39662,#32186,#32187);
#27237=AXIS2_PLACEMENT_3D('',#39666,#32190,#32191);
#27238=AXIS2_PLACEMENT_3D('',#39670,#32194,#32195);
#27239=AXIS2_PLACEMENT_3D('',#39674,#32198,#32199);
#27240=AXIS2_PLACEMENT_3D('',#39678,#32202,#32203);
#27241=AXIS2_PLACEMENT_3D('',#39684,#32207,#32208);
#27242=AXIS2_PLACEMENT_3D('',#39688,#32211,#32212);
#27243=AXIS2_PLACEMENT_3D('',#39692,#32215,#32216);
#27244=AXIS2_PLACEMENT_3D('',#39696,#32219,#32220);
#27245=AXIS2_PLACEMENT_3D('',#39700,#32223,#32224);
#27246=AXIS2_PLACEMENT_3D('',#39702,#32226,#32227);
#27247=AXIS2_PLACEMENT_3D('',#39703,#32228,#32229);
#27248=AXIS2_PLACEMENT_3D('',#39711,#32230,#32231);
#27249=AXIS2_PLACEMENT_3D('',#39719,#32232,#32233);
#27250=AXIS2_PLACEMENT_3D('',#39727,#32234,#32235);
#27251=AXIS2_PLACEMENT_3D('',#39735,#32236,#32237);
#27252=AXIS2_PLACEMENT_3D('',#39743,#32238,#32239);
#27253=AXIS2_PLACEMENT_3D('',#39751,#32240,#32241);
#27254=AXIS2_PLACEMENT_3D('',#39759,#32242,#32243);
#27255=AXIS2_PLACEMENT_3D('',#39767,#32244,#32245);
#27256=AXIS2_PLACEMENT_3D('',#39775,#32246,#32247);
#27257=AXIS2_PLACEMENT_3D('',#39783,#32248,#32249);
#27258=AXIS2_PLACEMENT_3D('',#39786,#32252,#32253);
#27259=AXIS2_PLACEMENT_3D('',#39788,#32255,#32256);
#27260=AXIS2_PLACEMENT_3D('',#39790,#32258,#32259);
#27261=AXIS2_PLACEMENT_3D('',#39792,#32261,#32262);
#27262=AXIS2_PLACEMENT_3D('',#39794,#32264,#32265);
#27263=AXIS2_PLACEMENT_3D('',#39795,#32266,#32267);
#32091=DIRECTION('axis',(0.,0.,1.));
#32092=DIRECTION('refdir',(1.,0.,0.));
#32093=DIRECTION('center_axis',(-6.99485272571294E-17,-0.923879532511288,
0.382683432365087));
#32094=DIRECTION('ref_axis',(0.,-0.382683432365087,-0.923879532511288));
#32095=DIRECTION('center_axis',(0.,0.923879532511288,-0.382683432365087));
#32096=DIRECTION('ref_axis',(0.,0.382683432365087,0.923879532511288));
#32097=DIRECTION('center_axis',(1.,-1.77588086089071E-17,1.39910753728411E-16));
#32098=DIRECTION('ref_axis',(-1.22464679914735E-16,0.382683432365087,0.923879532511288));
#32099=DIRECTION('center_axis',(-6.99485272571294E-17,-0.923879532511288,
0.382683432365087));
#32100=DIRECTION('ref_axis',(6.87413134363318E-33,-0.382683432365087,-0.923879532511288));
#32101=DIRECTION('center_axis',(-1.,1.77588086089071E-17,-1.39910753728411E-16));
#32102=DIRECTION('ref_axis',(-1.22464679914735E-16,0.382683432365087,0.923879532511288));
#32103=DIRECTION('center_axis',(-6.99485272571294E-17,-0.923879532511288,
0.382683432365087));
#32104=DIRECTION('ref_axis',(1.30371071656723E-32,-0.382683432365087,-0.923879532511288));
#32105=DIRECTION('center_axis',(-6.99485272571294E-17,-0.923879532511288,
0.382683432365087));
#32106=DIRECTION('ref_axis',(7.11155521594025E-34,-0.382683432365087,-0.923879532511288));
#32107=DIRECTION('',(1.0961176199419E-16,0.722104291896042,-0.691784208858019));
#32108=DIRECTION('center_axis',(-6.99485272571294E-17,-0.923879532511288,
0.382683432365087));
#32109=DIRECTION('ref_axis',(7.11155521594025E-34,-0.382683432365087,-0.923879532511288));
#32110=DIRECTION('center_axis',(-0.5,-0.33141357403559,-0.800103145191267));
#32111=DIRECTION('ref_axis',(-0.866025403784439,0.191341716182545,0.461939766255643));
#32112=DIRECTION('center_axis',(-6.99485272571294E-17,-0.923879532511288,
0.382683432365087));
#32113=DIRECTION('ref_axis',(-4.26190864642653E-32,-0.382683432365087,-0.923879532511288));
#32114=DIRECTION('center_axis',(0.,-0.923879532511288,0.382683432365087));
#32115=DIRECTION('ref_axis',(0.,-0.382683432365087,-0.923879532511288));
#32116=DIRECTION('center_axis',(0.,-0.923879532511288,0.382683432365087));
#32117=DIRECTION('ref_axis',(0.,-0.382683432365087,-0.923879532511288));
#32118=DIRECTION('center_axis',(0.,0.923879532511288,-0.382683432365087));
#32119=DIRECTION('ref_axis',(0.,0.382683432365087,0.923879532511288));
#32120=DIRECTION('center_axis',(0.,0.923879532511288,-0.382683432365087));
#32121=DIRECTION('ref_axis',(0.,0.382683432365087,0.923879532511288));
#32122=DIRECTION('center_axis',(0.,-0.923879532511288,0.382683432365087));
#32123=DIRECTION('ref_axis',(0.,-0.382683432365087,-0.923879532511288));
#32124=DIRECTION('center_axis',(0.,-0.923879532511288,0.382683432365087));
#32125=DIRECTION('ref_axis',(0.,-0.382683432365087,-0.923879532511288));
#32126=DIRECTION('',(0.,0.923879532511288,-0.382683432365087));
#32127=DIRECTION('center_axis',(0.,-0.923879532511288,0.382683432365087));
#32128=DIRECTION('ref_axis',(0.,-0.382683432365087,-0.923879532511288));
#32129=DIRECTION('center_axis',(0.,0.,-1.));
#32130=DIRECTION('ref_axis',(-1.,0.,0.));
#32131=DIRECTION('center_axis',(0.,0.,-1.));
#32132=DIRECTION('ref_axis',(-1.,0.,0.));
#32133=DIRECTION('center_axis',(0.,0.,-1.));
#32134=DIRECTION('ref_axis',(-1.,0.,0.));
#32135=DIRECTION('center_axis',(0.,0.,-1.));
#32136=DIRECTION('ref_axis',(-1.,0.,0.));
#32137=DIRECTION('',(0.,0.,1.));
#32138=DIRECTION('center_axis',(0.,0.,-1.));
#32139=DIRECTION('ref_axis',(-1.,0.,0.));
#32140=DIRECTION('center_axis',(0.,0.,-1.));
#32141=DIRECTION('ref_axis',(-1.,0.,0.));
#32142=DIRECTION('center_axis',(0.,0.,-1.));
#32143=DIRECTION('ref_axis',(-1.,0.,0.));
#32144=DIRECTION('center_axis',(0.,0.,-1.));
#32145=DIRECTION('ref_axis',(-1.,0.,0.));
#32146=DIRECTION('center_axis',(0.,0.,-1.));
#32147=DIRECTION('ref_axis',(-1.,0.,0.));
#32148=DIRECTION('center_axis',(0.,0.,-1.));
#32149=DIRECTION('ref_axis',(-1.,0.,0.));
#32150=DIRECTION('center_axis',(6.12323399573677E-17,0.,1.));
#32151=DIRECTION('ref_axis',(1.,0.,0.));
#32152=DIRECTION('center_axis',(1.22464679914735E-16,-1.,0.));
#32153=DIRECTION('ref_axis',(-1.,-1.22464679914735E-16,0.));
#32154=DIRECTION('center_axis',(0.,-0.923879532511288,0.382683432365087));
#32155=DIRECTION('ref_axis',(0.,-0.382683432365087,-0.923879532511288));
#32156=DIRECTION('center_axis',(0.,-0.923879532511288,0.382683432365087));
#32157=DIRECTION('ref_axis',(0.,-0.382683432365087,-0.923879532511288));
#32158=DIRECTION('center_axis',(0.,-0.923879532511288,0.382683432365087));
#32159=DIRECTION('ref_axis',(0.,-0.382683432365087,-0.923879532511288));
#32160=DIRECTION('center_axis',(0.,-0.923879532511288,0.382683432365087));
#32161=DIRECTION('ref_axis',(0.,-0.382683432365087,-0.923879532511288));
#32162=DIRECTION('center_axis',(0.,-0.923879532511288,0.382683432365087));
#32163=DIRECTION('ref_axis',(0.,-0.382683432365087,-0.923879532511288));
#32164=DIRECTION('center_axis',(0.,-0.923879532511288,0.382683432365087));
#32165=DIRECTION('ref_axis',(0.,-0.382683432365087,-0.923879532511288));
#32166=DIRECTION('center_axis',(0.,0.923879532511288,-0.382683432365087));
#32167=DIRECTION('ref_axis',(0.,0.382683432365087,0.923879532511288));
#32168=DIRECTION('center_axis',(0.,0.923879532511288,-0.382683432365087));
#32169=DIRECTION('ref_axis',(0.,0.382683432365087,0.923879532511288));
#32170=DIRECTION('center_axis',(0.,0.923879532511288,-0.382683432365087));
#32171=DIRECTION('ref_axis',(0.,0.382683432365087,0.923879532511288));
#32172=DIRECTION('center_axis',(0.,0.923879532511288,-0.382683432365087));
#32173=DIRECTION('ref_axis',(0.,0.382683432365087,0.923879532511288));
#32174=DIRECTION('center_axis',(0.,0.923879532511288,-0.382683432365087));
#32175=DIRECTION('ref_axis',(0.,0.382683432365087,0.923879532511288));
#32176=DIRECTION('center_axis',(0.,-0.923879532511288,0.382683432365087));
#32177=DIRECTION('ref_axis',(0.,-0.382683432365087,-0.923879532511288));
#32178=DIRECTION('center_axis',(0.,0.,1.));
#32179=DIRECTION('ref_axis',(1.,0.,0.));
#32180=DIRECTION('',(3.56799717200074E-15,-1.,0.));
#32181=DIRECTION('',(-0.866025403784438,-0.500000000000001,0.));
#32182=DIRECTION('center_axis',(0.,0.,1.));
#32183=DIRECTION('ref_axis',(1.,0.,0.));
#32184=DIRECTION('',(-0.866025403784438,-0.500000000000001,0.));
#32185=DIRECTION('',(-0.866025403784441,0.499999999999995,0.));
#32186=DIRECTION('center_axis',(0.,0.,1.));
#32187=DIRECTION('ref_axis',(1.,0.,0.));
#32188=DIRECTION('',(-0.866025403784441,0.499999999999995,0.));
#32189=DIRECTION('',(-1.05162021911601E-14,1.,0.));
#32190=DIRECTION('center_axis',(0.,0.,1.));
#32191=DIRECTION('ref_axis',(1.,0.,0.));
#32192=DIRECTION('',(-1.05162021911601E-14,1.,0.));
#32193=DIRECTION('',(0.866025403784434,0.500000000000007,0.));
#32194=DIRECTION('center_axis',(0.,0.,1.));
#32195=DIRECTION('ref_axis',(1.,0.,0.));
#32196=DIRECTION('',(0.866025403784434,0.500000000000007,0.));
#32197=DIRECTION('',(0.866025403784441,-0.499999999999995,0.));
#32198=DIRECTION('center_axis',(0.,0.,1.));
#32199=DIRECTION('ref_axis',(1.,0.,0.));
#32200=DIRECTION('',(0.866025403784441,-0.499999999999995,0.));
#32201=DIRECTION('',(3.56799717200074E-15,-1.,0.));
#32202=DIRECTION('center_axis',(0.499999999999995,0.866025403784442,0.));
#32203=DIRECTION('ref_axis',(-0.866025403784441,0.499999999999995,0.));
#32204=DIRECTION('',(-0.866025403784441,0.499999999999995,0.));
#32205=DIRECTION('',(0.,0.,1.));
#32206=DIRECTION('',(0.,0.,1.));
#32207=DIRECTION('center_axis',(1.,1.05162021911601E-14,0.));
#32208=DIRECTION('ref_axis',(-1.05162021911601E-14,1.,0.));
#32209=DIRECTION('',(-1.05162021911601E-14,1.,0.));
#32210=DIRECTION('',(0.,0.,1.));
#32211=DIRECTION('center_axis',(0.500000000000007,-0.866025403784435,0.));
#32212=DIRECTION('ref_axis',(0.866025403784435,0.500000000000007,0.));
#32213=DIRECTION('',(0.866025403784434,0.500000000000007,0.));
#32214=DIRECTION('',(0.,0.,1.));
#32215=DIRECTION('center_axis',(-0.499999999999995,-0.866025403784441,0.));
#32216=DIRECTION('ref_axis',(0.866025403784442,-0.499999999999995,0.));
#32217=DIRECTION('',(0.866025403784441,-0.499999999999995,0.));
#32218=DIRECTION('',(0.,0.,1.));
#32219=DIRECTION('center_axis',(-1.,-3.56799717200074E-15,0.));
#32220=DIRECTION('ref_axis',(3.56799717200074E-15,-1.,0.));
#32221=DIRECTION('',(3.56799717200074E-15,-1.,0.));
#32222=DIRECTION('',(0.,0.,1.));
#32223=DIRECTION('center_axis',(-0.500000000000001,0.866025403784438,0.));
#32224=DIRECTION('ref_axis',(-0.866025403784438,-0.500000000000001,0.));
#32225=DIRECTION('',(-0.866025403784438,-0.500000000000001,0.));
#32226=DIRECTION('center_axis',(0.,0.,1.));
#32227=DIRECTION('ref_axis',(1.,0.,0.));
#32228=DIRECTION('center_axis',(0.,0.923879532511288,-0.382683432365087));
#32229=DIRECTION('ref_axis',(0.,0.382683432365087,0.923879532511288));
#32230=DIRECTION('center_axis',(0.,0.923879532511288,-0.382683432365087));
#32231=DIRECTION('ref_axis',(0.,0.382683432365087,0.923879532511288));
#32232=DIRECTION('center_axis',(0.,0.923879532511288,-0.382683432365087));
#32233=DIRECTION('ref_axis',(1.22464679914735E-16,-0.382683432365087,-0.923879532511288));
#32234=DIRECTION('center_axis',(0.,0.923879532511288,-0.382683432365087));
#32235=DIRECTION('ref_axis',(0.,0.382683432365087,0.923879532511288));
#32236=DIRECTION('center_axis',(0.,0.923879532511288,-0.382683432365087));
#32237=DIRECTION('ref_axis',(0.,0.382683432365087,0.923879532511288));
#32238=DIRECTION('center_axis',(0.,-0.923879532511288,0.382683432365087));
#32239=DIRECTION('ref_axis',(0.,-0.382683432365087,-0.923879532511288));
#32240=DIRECTION('center_axis',(0.,-0.923879532511288,0.382683432365087));
#32241=DIRECTION('ref_axis',(0.,-0.382683432365087,-0.923879532511288));
#32242=DIRECTION('center_axis',(0.,-0.923879532511288,0.382683432365087));
#32243=DIRECTION('ref_axis',(-7.6571373978539E-16,0.382683432365087,0.923879532511288));
#32244=DIRECTION('center_axis',(0.,-0.923879532511288,0.382683432365087));
#32245=DIRECTION('ref_axis',(0.,-0.382683432365087,-0.923879532511288));
#32246=DIRECTION('center_axis',(0.,-0.923879532511288,0.382683432365087));
#32247=DIRECTION('ref_axis',(0.,-0.382683432365087,-0.923879532511288));
#32248=DIRECTION('center_axis',(-0.5,-0.331413574035589,-0.800103145191266));
#32249=DIRECTION('ref_axis',(-0.84802901144343,6.89411318440465E-18,0.529949804934655));
#32250=DIRECTION('',(0.,0.923879532511288,-0.382683432365087));
#32251=DIRECTION('',(0.,0.923879532511288,-0.382683432365087));
#32252=DIRECTION('center_axis',(-1.,4.14906208744436E-17,1.00167219626363E-16));
#32253=DIRECTION('ref_axis',(1.00167219626363E-16,0.,1.));
#32254=DIRECTION('',(0.,0.923879532511288,-0.382683432365087));
#32255=DIRECTION('center_axis',(-0.5,0.331413574035589,0.800103145191267));
#32256=DIRECTION('ref_axis',(0.848029011443431,-1.03411697766071E-17,0.529949804934654));
#32257=DIRECTION('',(0.,0.923879532511288,-0.382683432365087));
#32258=DIRECTION('center_axis',(0.5,0.331413574035589,0.800103145191267));
#32259=DIRECTION('ref_axis',(0.84802901144343,-3.44705659220234E-18,-0.529949804934655));
#32260=DIRECTION('',(0.,0.923879532511288,-0.382683432365087));
#32261=DIRECTION('center_axis',(1.,0.,0.));
#32262=DIRECTION('ref_axis',(0.,0.,-1.));
#32263=DIRECTION('',(0.,0.923879532511288,-0.382683432365087));
#32264=DIRECTION('center_axis',(0.499999999999999,-0.33141357403559,-0.800103145191267));
#32265=DIRECTION('ref_axis',(-0.848029011443431,5.08102344929861E-18,-0.529949804934654));
#32266=DIRECTION('center_axis',(-6.99485272571294E-17,-0.923879532511288,
0.382683432365087));
#32267=DIRECTION('ref_axis',(-2.37033238942555E-33,-0.382683432365087,-0.923879532511288));
#39518=CARTESIAN_POINT('',(0.,0.,0.));
#39519=CARTESIAN_POINT('Origin',(-1.30104260698261E-15,5.62313017679403,
-9.43017678221748));
#39520=CARTESIAN_POINT('',(-9.42566476249075E-16,6.10854241414471,-5.90647463868609));
#39521=CARTESIAN_POINT('Origin',(-1.30104260698261E-15,4.79163859753386,
-9.0857616930889));
#39522=CARTESIAN_POINT('',(-1.65091236461116E-15,7.42947410803995,-6.70023456114395));
#39523=CARTESIAN_POINT('Origin',(-1.82151749662023E-15,7.24953476434565,
-5.50368876904451));
#39524=CARTESIAN_POINT('Origin',(-1.1944312217556E-15,6.1997608355023,-9.66902502153458));
#39525=CARTESIAN_POINT('Ctrl Pts',(-1.0334492107102E-15,9.1104629285565,
-7.23378761718564));
#39526=CARTESIAN_POINT('Ctrl Pts',(-3.36374346224613,9.1104629285565,-7.23378761718564));
#39527=CARTESIAN_POINT('Ctrl Pts',(-3.36374346224613,7.82321403482853,-10.3414813545735));
#39528=CARTESIAN_POINT('Ctrl Pts',(-3.36374346224613,6.53596514110056,-13.4491750919613));
#39529=CARTESIAN_POINT('Ctrl Pts',(-1.0334492107102E-15,6.53596514110056,
-13.4491750919613));
#39530=CARTESIAN_POINT('Ctrl Pts',(3.36374346224612,6.53596514110056,-13.4491750919613));
#39531=CARTESIAN_POINT('Ctrl Pts',(3.36374346224612,7.82321403482853,-10.3414813545735));
#39532=CARTESIAN_POINT('Ctrl Pts',(3.36374346224612,9.1104629285565,-7.23378761718564));
#39533=CARTESIAN_POINT('Ctrl Pts',(-1.0334492107102E-15,9.1104629285565,
-7.23378761718564));
#39534=CARTESIAN_POINT('Ctrl Pts',(-1.09748950322703E-15,8.40101827381132,
-6.55413148618164));
#39535=CARTESIAN_POINT('Ctrl Pts',(-3.72017113527558,8.40101827381132,-6.55413148618164));
#39536=CARTESIAN_POINT('Ctrl Pts',(-3.72017113527558,6.97737041477854,-9.99112145550203));
#39537=CARTESIAN_POINT('Ctrl Pts',(-3.72017113527558,5.55372255574576,-13.4281114248224));
#39538=CARTESIAN_POINT('Ctrl Pts',(-1.09748950322703E-15,5.55372255574576,
-13.4281114248224));
#39539=CARTESIAN_POINT('Ctrl Pts',(3.72017113527558,5.55372255574576,-13.4281114248224));
#39540=CARTESIAN_POINT('Ctrl Pts',(3.72017113527558,6.97737041477854,-9.99112145550203));
#39541=CARTESIAN_POINT('Ctrl Pts',(3.72017113527558,8.40101827381132,-6.55413148618164));
#39542=CARTESIAN_POINT('Ctrl Pts',(-1.09748950322703E-15,8.40101827381132,
-6.55413148618164));
#39543=CARTESIAN_POINT('Ctrl Pts',(-1.15636367776747E-15,7.42947410803995,
-6.70023456114395));
#39544=CARTESIAN_POINT('Ctrl Pts',(-3.21339563862928,7.42947410803995,-6.70023456114395));
#39545=CARTESIAN_POINT('Ctrl Pts',(-3.21339563862928,6.1997608355023,-9.66902502153458));
#39546=CARTESIAN_POINT('Ctrl Pts',(-3.21339563862928,4.97004756296464,-12.6378154819252));
#39547=CARTESIAN_POINT('Ctrl Pts',(-1.15636367776747E-15,4.97004756296464,
-12.6378154819252));
#39548=CARTESIAN_POINT('Ctrl Pts',(3.21339563862928,4.97004756296464,-12.6378154819252));
#39549=CARTESIAN_POINT('Ctrl Pts',(3.21339563862928,6.1997608355023,-9.66902502153458));
#39550=CARTESIAN_POINT('Ctrl Pts',(3.21339563862928,7.42947410803995,-6.70023456114395));
#39551=CARTESIAN_POINT('Ctrl Pts',(-1.15636367776747E-15,7.42947410803995,
-6.70023456114395));
#39552=CARTESIAN_POINT('',(-1.44538897712945E-15,9.1104629285565,-7.23378761718564));
#39553=CARTESIAN_POINT('Origin',(-1.26789919235761E-15,7.72689451084046,
-8.67799620097772));
#39554=CARTESIAN_POINT('Origin',(-1.07151675469833E-15,7.82321403482853,
-10.3414813545735));
#39555=CARTESIAN_POINT('Origin',(-9.16325707068394E-16,9.87297602634596,
-11.1905205710969));
#39556=CARTESIAN_POINT('',(-1.22248740685523E-15,10.8296846072587,-8.88082173981866));
#39557=CARTESIAN_POINT('',(-1.22248740685523E-15,10.8296846072587,-8.88082173981866));
#39558=CARTESIAN_POINT('Origin',(-9.16325707068394E-16,9.87297602634596,
-11.1905205710969));
#39559=CARTESIAN_POINT('Origin',(-8.67361737988404E-16,9.41103626009031,
-10.9991788549143));
#39560=CARTESIAN_POINT('',(0.944722181384557,9.66424685661039,-11.6944373635354));
#39561=CARTESIAN_POINT('Origin',(-9.16325707068394E-16,9.87297602634596,
-11.1905205710969));
#39562=CARTESIAN_POINT('Origin',(0.,4.50578927537974,-8.96735902705751));
#39563=CARTESIAN_POINT('',(-1.73205080756888,3.64358830043861,-11.8574002906228));
#39564=CARTESIAN_POINT('',(1.73205080756888,3.64358830043861,-11.8574002906228));
#39565=CARTESIAN_POINT('Origin',(0.,4.79163859753386,-9.08576169308891));
#39566=CARTESIAN_POINT('',(-8.67361737988404E-16,2.97505554591939,-12.6628771571027));
#39567=CARTESIAN_POINT('Ctrl Pts',(-8.83559534733916E-12,2.97505554591472,
-12.6628771571063));
#39568=CARTESIAN_POINT('Ctrl Pts',(0.928203230271955,3.46598430139072,-12.2861742738559));
#39569=CARTESIAN_POINT('Ctrl Pts',(1.73205080756887,3.6435883004386,-11.8574002906228));
#39570=CARTESIAN_POINT('Ctrl Pts',(-1.73205080756888,3.64358830043861,-11.8574002906228));
#39571=CARTESIAN_POINT('Ctrl Pts',(-0.928203230271849,3.46598430139071,
-12.2861742738559));
#39572=CARTESIAN_POINT('Ctrl Pts',(9.11080614203771E-12,2.97505554591457,
-12.6628771571064));
#39573=CARTESIAN_POINT('Origin',(0.,2.94387953251129,-8.32039482835873));
#39574=CARTESIAN_POINT('',(-1.73205080756888,4.09192982960656,-5.54875623082487));
#39575=CARTESIAN_POINT('',(1.73205080756888,4.09192982960656,-5.54875623082487));
#39576=CARTESIAN_POINT('Origin',(0.,2.94387953251129,-8.32039482835873));
#39577=CARTESIAN_POINT('',(6.50521303491303E-15,4.76046258412578,-4.74327936434497));
#39578=CARTESIAN_POINT('Ctrl Pts',(-8.84140945978337E-12,4.76046258413045,
-4.74327936434139));
#39579=CARTESIAN_POINT('Ctrl Pts',(0.928203230271958,4.26953382865444,-5.11998224759177));
#39580=CARTESIAN_POINT('Ctrl Pts',(1.73205080756888,4.09192982960656,-5.54875623082487));
#39581=CARTESIAN_POINT('Ctrl Pts',(-1.73205080756888,4.09192982960655,-5.54875623082487));
#39582=CARTESIAN_POINT('Ctrl Pts',(-0.928203230271845,4.26953382865446,
-5.11998224759171));
#39583=CARTESIAN_POINT('Ctrl Pts',(9.11907870314464E-12,4.7604625841306,
-4.74327936434127));
#39584=CARTESIAN_POINT('Origin',(0.,0.,-7.101));
#39585=CARTESIAN_POINT('',(-2.79266716119615,2.86374058300968,-7.101));
#39586=CARTESIAN_POINT('',(2.79266716119615,2.86374058300968,-7.101));
#39587=CARTESIAN_POINT('Origin',(0.,2.44435548440748,-8.11348519290263));
#39588=CARTESIAN_POINT('',(-4.61252776028392E-16,4.,-5.51067764861519));
#39589=CARTESIAN_POINT('Ctrl Pts',(-2.79266716119614,2.86374058300969,-7.10099999999999));
#39590=CARTESIAN_POINT('Ctrl Pts',(-2.791487395233,2.86489106908469,-7.0982224809144));
#39591=CARTESIAN_POINT('Ctrl Pts',(-2.79030270745925,2.86604495955758,-7.09544824938184));
#39592=CARTESIAN_POINT('Ctrl Pts',(-2.64444489381139,3.00792702197672,-6.75569806071638));
#39593=CARTESIAN_POINT('Ctrl Pts',(-2.42146694806281,3.19843151589414,-6.46722664985982));
#39594=CARTESIAN_POINT('Ctrl Pts',(-1.897815678339,3.53535819041829,-6.01625804314877));
#39595=CARTESIAN_POINT('Ctrl Pts',(-1.5580225174343,3.70511768616704,-5.82557882438308));
#39596=CARTESIAN_POINT('Ctrl Pts',(-0.804950314595278,3.93794187104499,
-5.57277579859251));
#39597=CARTESIAN_POINT('Ctrl Pts',(-0.391351836138015,4.,-5.51067764861519));
#39598=CARTESIAN_POINT('Ctrl Pts',(-3.46944695195361E-16,4.,-5.51067764861519));
#39599=CARTESIAN_POINT('',(-3.67394039744206E-16,4.09192982960655,-5.54875623082487));
#39600=CARTESIAN_POINT('',(-3.67394039744206E-16,1.14805029709526,-4.32936140246614));
#39601=CARTESIAN_POINT('Origin',(0.,2.94387953251129,-8.32039482835873));
#39602=CARTESIAN_POINT('Ctrl Pts',(-5.55111512312578E-16,4.,-5.51067764861519));
#39603=CARTESIAN_POINT('Ctrl Pts',(0.391351836138015,4.,-5.51067764861519));
#39604=CARTESIAN_POINT('Ctrl Pts',(0.804950314595278,3.93794187104499,-5.57277579859251));
#39605=CARTESIAN_POINT('Ctrl Pts',(1.5580225174343,3.70511768616704,-5.82557882438308));
#39606=CARTESIAN_POINT('Ctrl Pts',(1.897815678339,3.53535819041829,-6.01625804314877));
#39607=CARTESIAN_POINT('Ctrl Pts',(2.42146694806282,3.19843151589414,-6.46722664985983));
#39608=CARTESIAN_POINT('Ctrl Pts',(2.64444489381139,3.00792702197672,-6.75569806071639));
#39609=CARTESIAN_POINT('Ctrl Pts',(2.79030270745925,2.86604495955758,-7.09544824938184));
#39610=CARTESIAN_POINT('Ctrl Pts',(2.791487395233,2.86489106908469,-7.0982224809144));
#39611=CARTESIAN_POINT('Ctrl Pts',(2.79266716119614,2.86374058300969,-7.10099999999999));
#39612=CARTESIAN_POINT('Origin',(0.,0.,-13.5441803724939));
#39613=CARTESIAN_POINT('',(4.,-4.89858719658941E-16,-7.101));
#39614=CARTESIAN_POINT('Origin',(0.,0.,-7.101));
#39615=CARTESIAN_POINT('',(-4.,-4.89858719658941E-16,-7.101));
#39616=CARTESIAN_POINT('Origin',(0.,0.,-7.101));
#39617=CARTESIAN_POINT('Origin',(0.,0.,-7.101));
#39618=CARTESIAN_POINT('',(4.,4.20648087646404E-14,-3.));
#39619=CARTESIAN_POINT('',(4.,-4.89858719658941E-16,-13.5441803724939));
#39620=CARTESIAN_POINT('',(2.00000000000003,-3.46410161513774,-3.));
#39621=CARTESIAN_POINT('Origin',(0.,0.,-3.));
#39622=CARTESIAN_POINT('',(-1.99999999999998,-3.46410161513777,-3.));
#39623=CARTESIAN_POINT('Origin',(0.,0.,-3.));
#39624=CARTESIAN_POINT('',(-4.,-1.4271988688003E-14,-3.));
#39625=CARTESIAN_POINT('Origin',(0.,0.,-3.));
#39626=CARTESIAN_POINT('',(-2.,3.46410161513775,-3.));
#39627=CARTESIAN_POINT('Origin',(0.,0.,-3.));
#39628=CARTESIAN_POINT('',(1.99999999999999,3.46410161513778,-3.));
#39629=CARTESIAN_POINT('Origin',(0.,0.,-3.));
#39630=CARTESIAN_POINT('Origin',(0.,0.,-3.));
#39631=CARTESIAN_POINT('Origin',(0.,0.,-7.101));
#39632=CARTESIAN_POINT('',(-2.44929359829471E-16,-2.99951956532372E-32,
-11.101));
#39633=CARTESIAN_POINT('Origin',(0.,0.,-7.101));
#39634=CARTESIAN_POINT('Origin',(0.,6.32237232699421,-5.39024356304375));
#39635=CARTESIAN_POINT('',(3.46410161513776,4.79163859753387,-9.08576169308891));
#39636=CARTESIAN_POINT('Origin',(0.,4.79163859753387,-9.08576169308891));
#39637=CARTESIAN_POINT('',(-3.46410161513776,4.79163859753387,-9.08576169308891));
#39638=CARTESIAN_POINT('Origin',(0.,4.79163859753386,-9.08576169308891));
#39639=CARTESIAN_POINT('',(-1.73205080756888,5.93968889462913,-6.31412309555504));
#39640=CARTESIAN_POINT('Origin',(0.,4.79163859753386,-9.08576169308891));
#39641=CARTESIAN_POINT('',(1.73205080756888,5.93968889462913,-6.31412309555504));
#39642=CARTESIAN_POINT('Origin',(0.,4.79163859753386,-9.08576169308891));
#39643=CARTESIAN_POINT('Origin',(0.,4.79163859753386,-9.08576169308891));
#39644=CARTESIAN_POINT('Origin',(0.,4.47461326197163,-4.62487669831358));
#39645=CARTESIAN_POINT('',(3.46410161513776,2.94387953251129,-8.32039482835873));
#39646=CARTESIAN_POINT('Origin',(0.,2.94387953251129,-8.32039482835873));
#39647=CARTESIAN_POINT('',(-3.46410161513776,2.94387953251129,-8.32039482835873));
#39648=CARTESIAN_POINT('Origin',(0.,2.94387953251129,-8.32039482835873));
#39649=CARTESIAN_POINT('',(-1.73205080756888,1.79582923541603,-11.0920334258926));
#39650=CARTESIAN_POINT('Origin',(0.,2.94387953251129,-8.32039482835873));
#39651=CARTESIAN_POINT('',(1.73205080756888,1.79582923541603,-11.0920334258926));
#39652=CARTESIAN_POINT('Origin',(0.,2.94387953251129,-8.32039482835873));
#39653=CARTESIAN_POINT('Origin',(0.,2.94387953251129,-8.32039482835873));
#39654=CARTESIAN_POINT('Origin',(0.,0.,-3.));
#39655=CARTESIAN_POINT('',(-4.00000000000001,2.3094010767585,-3.));
#39656=CARTESIAN_POINT('',(-4.00000000000001,2.3094010767585,-3.));
#39657=CARTESIAN_POINT('',(0.,4.61880215351701,-3.));
#39658=CARTESIAN_POINT('Origin',(0.,0.,-3.));
#39659=CARTESIAN_POINT('',(0.,4.61880215351701,-3.));
#39660=CARTESIAN_POINT('',(0.,4.61880215351701,-3.));
#39661=CARTESIAN_POINT('',(3.99999999999998,2.30940107675855,-3.));
#39662=CARTESIAN_POINT('Origin',(0.,0.,-3.));
#39663=CARTESIAN_POINT('',(3.99999999999998,2.30940107675855,-3.));
#39664=CARTESIAN_POINT('',(3.99999999999998,2.30940107675855,-3.));
#39665=CARTESIAN_POINT('',(4.00000000000002,-2.30940107675847,-3.));
#39666=CARTESIAN_POINT('Origin',(0.,0.,-3.));
#39667=CARTESIAN_POINT('',(4.00000000000002,-2.30940107675847,-3.));
#39668=CARTESIAN_POINT('',(4.00000000000002,-2.30940107675847,-3.));
#39669=CARTESIAN_POINT('',(3.22529230536262E-14,-4.61880215351701,-3.));
#39670=CARTESIAN_POINT('Origin',(0.,0.,-3.));
#39671=CARTESIAN_POINT('',(3.22529230536262E-14,-4.61880215351701,-3.));
#39672=CARTESIAN_POINT('',(3.22529230536262E-14,-4.61880215351701,-3.));
#39673=CARTESIAN_POINT('',(-3.99999999999999,-2.30940107675852,-3.));
#39674=CARTESIAN_POINT('Origin',(0.,0.,-3.));
#39675=CARTESIAN_POINT('',(-3.99999999999999,-2.30940107675852,-3.));
#39676=CARTESIAN_POINT('',(-3.99999999999999,-2.30940107675852,-3.));
#39677=CARTESIAN_POINT('',(-4.00000000000001,2.3094010767585,-3.));
#39678=CARTESIAN_POINT('Origin',(3.99999999999998,2.30940107675855,-3.));
#39679=CARTESIAN_POINT('',(3.99999999999998,2.30940107675855,0.));
#39680=CARTESIAN_POINT('',(0.,4.61880215351701,0.));
#39681=CARTESIAN_POINT('',(3.99999999999998,2.30940107675855,0.));
#39682=CARTESIAN_POINT('',(3.99999999999998,2.30940107675855,-3.));
#39683=CARTESIAN_POINT('',(0.,4.61880215351701,-3.));
#39684=CARTESIAN_POINT('Origin',(4.00000000000002,-2.30940107675847,-3.));
#39685=CARTESIAN_POINT('',(4.00000000000002,-2.30940107675847,0.));
#39686=CARTESIAN_POINT('',(4.00000000000002,-2.30940107675847,0.));
#39687=CARTESIAN_POINT('',(4.00000000000002,-2.30940107675847,-3.));
#39688=CARTESIAN_POINT('Origin',(3.22529230536262E-14,-4.61880215351701,
-3.));
#39689=CARTESIAN_POINT('',(3.22529230536262E-14,-4.61880215351701,0.));
#39690=CARTESIAN_POINT('',(3.22529230536262E-14,-4.61880215351701,0.));
#39691=CARTESIAN_POINT('',(3.22529230536262E-14,-4.61880215351701,-3.));
#39692=CARTESIAN_POINT('Origin',(-3.99999999999999,-2.30940107675852,-3.));
#39693=CARTESIAN_POINT('',(-3.99999999999999,-2.30940107675852,0.));
#39694=CARTESIAN_POINT('',(-3.99999999999999,-2.30940107675852,0.));
#39695=CARTESIAN_POINT('',(-3.99999999999999,-2.30940107675852,-3.));
#39696=CARTESIAN_POINT('Origin',(-4.00000000000001,2.3094010767585,-3.));
#39697=CARTESIAN_POINT('',(-4.00000000000001,2.3094010767585,0.));
#39698=CARTESIAN_POINT('',(-4.00000000000001,2.3094010767585,0.));
#39699=CARTESIAN_POINT('',(-4.00000000000001,2.3094010767585,-3.));
#39700=CARTESIAN_POINT('Origin',(0.,4.61880215351701,-3.));
#39701=CARTESIAN_POINT('',(0.,4.61880215351701,0.));
#39702=CARTESIAN_POINT('Origin',(0.,0.,0.));
#39703=CARTESIAN_POINT('Origin',(0.,2.94387953251129,-8.32039482835873));
#39704=CARTESIAN_POINT('',(-3.46410161513776,3.9950957193956,-6.59103842936755));
#39705=CARTESIAN_POINT('Ctrl Pts',(-3.46410161513776,2.94387953251129,-8.32039482835873));
#39706=CARTESIAN_POINT('Ctrl Pts',(-3.46410161513776,3.29908753061063,-7.46284686188391));
#39707=CARTESIAN_POINT('Ctrl Pts',(-3.46410161513776,3.99509571941731,-6.59103842934036));
#39708=CARTESIAN_POINT('Ctrl Pts',(-3.46410161515884,3.99509571939744,-6.59103842938149));
#39709=CARTESIAN_POINT('Ctrl Pts',(-2.53589838487072,3.91432583055759,-5.97753021406059));
#39710=CARTESIAN_POINT('Ctrl Pts',(-1.73205080756888,4.09192982960655,-5.54875623082487));
#39711=CARTESIAN_POINT('Origin',(0.,2.94387953251129,-8.32039482835873));
#39712=CARTESIAN_POINT('',(-3.46410161513776,2.46436198993525,-10.2865565594127));
#39713=CARTESIAN_POINT('Ctrl Pts',(-1.73205080756888,1.79582923541603,-11.0920334258926));
#39714=CARTESIAN_POINT('Ctrl Pts',(-2.53589838486591,1.97343323446393,-10.6632594426594));
#39715=CARTESIAN_POINT('Ctrl Pts',(-3.46410161514687,2.46436198994007,-10.286556559409));
#39716=CARTESIAN_POINT('Ctrl Pts',(-3.46410161513776,2.46436198993072,-10.2865565594531));
#39717=CARTESIAN_POINT('Ctrl Pts',(-3.46410161513776,2.58867153441109,-9.17794279483566));
#39718=CARTESIAN_POINT('Ctrl Pts',(-3.46410161513776,2.94387953251129,-8.32039482835874));
#39719=CARTESIAN_POINT('Origin',(0.,2.94387953251129,-8.32039482835873));
#39720=CARTESIAN_POINT('',(3.90312782094782E-15,1.69899512520508,-12.1343156244353));
#39721=CARTESIAN_POINT('Ctrl Pts',(9.12142465330762E-12,1.69899512520587,
-12.1343156244413));
#39722=CARTESIAN_POINT('Ctrl Pts',(-0.928203230271842,1.61822523636812,
-11.5208074091258));
#39723=CARTESIAN_POINT('Ctrl Pts',(-1.73205080756888,1.79582923541603,-11.0920334258926));
#39724=CARTESIAN_POINT('Ctrl Pts',(1.73205080756888,1.79582923541603,-11.0920334258926));
#39725=CARTESIAN_POINT('Ctrl Pts',(0.928203230271956,1.61822523636815,-11.5208074091257));
#39726=CARTESIAN_POINT('Ctrl Pts',(-8.8435124366233E-12,1.69899512520584,
-12.1343156244411));
#39727=CARTESIAN_POINT('Origin',(0.,2.94387953251129,-8.32039482835873));
#39728=CARTESIAN_POINT('',(3.46410161513776,2.46436198993525,-10.2865565594127));
#39729=CARTESIAN_POINT('Ctrl Pts',(3.46410161514661,2.46436198993993,-10.2865565594091));
#39730=CARTESIAN_POINT('Ctrl Pts',(2.53589838486581,1.97343323446391,-10.6632594426595));
#39731=CARTESIAN_POINT('Ctrl Pts',(1.73205080756888,1.79582923541603,-11.0920334258926));
#39732=CARTESIAN_POINT('Ctrl Pts',(3.46410161513776,2.94387953251129,-8.32039482835873));
#39733=CARTESIAN_POINT('Ctrl Pts',(3.46410161513776,2.58867153441108,-9.17794279483565));
#39734=CARTESIAN_POINT('Ctrl Pts',(3.46410161513776,2.46436198993072,-10.2865565594531));
#39735=CARTESIAN_POINT('Origin',(0.,2.94387953251129,-8.32039482835873));
#39736=CARTESIAN_POINT('',(3.46410161513776,3.9950957193956,-6.59103842936756));
#39737=CARTESIAN_POINT('Ctrl Pts',(3.46410161513776,3.99509571941731,-6.59103842934036));
#39738=CARTESIAN_POINT('Ctrl Pts',(3.46410161513776,3.29908753061063,-7.46284686188391));
#39739=CARTESIAN_POINT('Ctrl Pts',(3.46410161513776,2.94387953251129,-8.32039482835873));
#39740=CARTESIAN_POINT('Ctrl Pts',(1.73205080756888,4.09192982960655,-5.54875623082487));
#39741=CARTESIAN_POINT('Ctrl Pts',(2.53589838487052,3.91432583055763,-5.97753021406048));
#39742=CARTESIAN_POINT('Ctrl Pts',(3.46410161515834,3.99509571939739,-6.59103842938115));
#39743=CARTESIAN_POINT('Origin',(0.,4.50578927537974,-8.96735902705751));
#39744=CARTESIAN_POINT('',(3.46410161513776,3.74042241064956,-10.8151180920801));
#39745=CARTESIAN_POINT('Ctrl Pts',(3.46410161513776,3.74042241062786,-10.8151180921073));
#39746=CARTESIAN_POINT('Ctrl Pts',(3.46410161513776,4.43643059943453,-9.94330965956373));
#39747=CARTESIAN_POINT('Ctrl Pts',(3.46410161513776,4.79163859753386,-9.08576169308893));
#39748=CARTESIAN_POINT('Ctrl Pts',(1.73205080756889,3.64358830043861,-11.8574002906228));
#39749=CARTESIAN_POINT('Ctrl Pts',(2.53589838487114,3.82119229948767,-11.4286263073868));
#39750=CARTESIAN_POINT('Ctrl Pts',(3.46410161515986,3.74042241064764,-10.8151180920655));
#39751=CARTESIAN_POINT('Origin',(0.,4.50578927537974,-8.96735902705751));
#39752=CARTESIAN_POINT('',(3.46410161513776,5.27115614010992,-7.11959996203494));
#39753=CARTESIAN_POINT('Ctrl Pts',(3.46410161514743,5.2711561401048,-7.11959996203886));
#39754=CARTESIAN_POINT('Ctrl Pts',(2.53589838486614,5.76208489558118,-6.74289707878832));
#39755=CARTESIAN_POINT('Ctrl Pts',(1.73205080756888,5.93968889462914,-6.31412309555504));
#39756=CARTESIAN_POINT('Ctrl Pts',(3.46410161513776,4.79163859753387,-9.08576169308891));
#39757=CARTESIAN_POINT('Ctrl Pts',(3.46410161513776,5.14684659563408,-8.22821372661199));
#39758=CARTESIAN_POINT('Ctrl Pts',(3.46410161513776,5.27115614011445,-7.11959996199452));
#39759=CARTESIAN_POINT('Origin',(0.,4.50578927537974,-8.96735902705751));
#39760=CARTESIAN_POINT('',(6.50521303491303E-15,6.03652300484009,-5.27184089701236));
#39761=CARTESIAN_POINT('Ctrl Pts',(9.66462909312592E-12,6.03652300483925,
-5.27184089700597));
#39762=CARTESIAN_POINT('Ctrl Pts',(-0.928203230271627,6.11729289367709,
-5.88534911232177));
#39763=CARTESIAN_POINT('Ctrl Pts',(-1.73205080756888,5.93968889462913,-6.31412309555505));
#39764=CARTESIAN_POINT('Ctrl Pts',(1.73205080756888,5.93968889462914,-6.31412309555504));
#39765=CARTESIAN_POINT('Ctrl Pts',(0.928203230271628,6.11729289367709,-5.88534911232177));
#39766=CARTESIAN_POINT('Ctrl Pts',(-9.6577405477995E-12,6.03652300483925,
-5.27184089700597));
#39767=CARTESIAN_POINT('Origin',(0.,4.50578927537974,-8.96735902705751));
#39768=CARTESIAN_POINT('',(-3.46410161513776,5.27115614010992,-7.11959996203493));
#39769=CARTESIAN_POINT('Ctrl Pts',(-3.46410161513776,5.27115614011445,-7.1195999619945));
#39770=CARTESIAN_POINT('Ctrl Pts',(-3.46410161513776,5.14684659563408,-8.22821372661199));
#39771=CARTESIAN_POINT('Ctrl Pts',(-3.46410161513776,4.79163859753387,-9.08576169308891));
#39772=CARTESIAN_POINT('Ctrl Pts',(-1.73205080756888,5.93968889462913,-6.31412309555505));
#39773=CARTESIAN_POINT('Ctrl Pts',(-2.53589838486613,5.76208489558118,-6.74289707878832));
#39774=CARTESIAN_POINT('Ctrl Pts',(-3.46410161514742,5.27115614010481,-7.11959996203885));
#39775=CARTESIAN_POINT('Origin',(0.,4.50578927537974,-8.96735902705751));
#39776=CARTESIAN_POINT('',(-3.46410161513776,3.74042241064957,-10.8151180920801));
#39777=CARTESIAN_POINT('Ctrl Pts',(-3.46410161515986,3.74042241064764,-10.8151180920655));
#39778=CARTESIAN_POINT('Ctrl Pts',(-2.53589838487113,3.82119229948767,-11.4286263073868));
#39779=CARTESIAN_POINT('Ctrl Pts',(-1.73205080756889,3.64358830043861,-11.8574002906228));
#39780=CARTESIAN_POINT('Ctrl Pts',(-3.46410161513776,4.79163859753387,-9.08576169308891));
#39781=CARTESIAN_POINT('Ctrl Pts',(-3.46410161513776,4.43643059943453,-9.94330965956373));
#39782=CARTESIAN_POINT('Ctrl Pts',(-3.46410161513776,3.74042241062786,-10.8151180921073));
#39783=CARTESIAN_POINT('Origin',(-8.67361737988404E-16,1.41314580305094,
-12.0159129584039));
#39784=CARTESIAN_POINT('',(-8.67361737988404E-16,1.41314580305094,-12.0159129584039));
#39785=CARTESIAN_POINT('',(-3.46410161513776,2.17851266778112,-10.1681538933813));
#39786=CARTESIAN_POINT('Origin',(-3.46410161513776,2.17851266778112,-10.1681538933813));
#39787=CARTESIAN_POINT('',(-3.46410161513776,3.70924639724147,-6.47263576333616));
#39788=CARTESIAN_POINT('Origin',(-3.46410161513776,3.70924639724147,-6.47263576333616));
#39789=CARTESIAN_POINT('',(7.02214595811131E-16,4.47461326197164,-4.62487669831358));
#39790=CARTESIAN_POINT('Origin',(7.02214595811131E-16,4.47461326197164,
-4.62487669831358));
#39791=CARTESIAN_POINT('',(3.46410161513776,3.70924639724147,-6.47263576333616));
#39792=CARTESIAN_POINT('Origin',(3.46410161513776,3.70924639724147,-6.47263576333616));
#39793=CARTESIAN_POINT('',(3.46410161513776,2.17851266778112,-10.1681538933813));
#39794=CARTESIAN_POINT('Origin',(3.46410161513776,2.17851266778112,-10.1681538933813));
#39795=CARTESIAN_POINT('Origin',(0.944722181384557,9.66424685661038,-11.6944373635354));
#66652=UNCERTAINTY_MEASURE_WITH_UNIT(LENGTH_MEASURE(0.01),#66722,
'DISTANCE_ACCURACY_VALUE',
'Maximum model space distance between geometric entities at asserted c
onnectivities');
#66680=UNCERTAINTY_MEASURE_WITH_UNIT(LENGTH_MEASURE(0.01),#66722,
'DISTANCE_ACCURACY_VALUE',
'Maximum model space distance between geometric entities at asserted c
onnectivities');
#66693=(
GEOMETRIC_REPRESENTATION_CONTEXT(3)
GLOBAL_UNCERTAINTY_ASSIGNED_CONTEXT((#66652))
GLOBAL_UNIT_ASSIGNED_CONTEXT((#66722,#66724,#66725))
REPRESENTATION_CONTEXT('','3D')
);
#66721=(
GEOMETRIC_REPRESENTATION_CONTEXT(3)
GLOBAL_UNCERTAINTY_ASSIGNED_CONTEXT((#66680))
GLOBAL_UNIT_ASSIGNED_CONTEXT((#66722,#66724,#66725))
REPRESENTATION_CONTEXT('','3D')
);
#66722=(
LENGTH_UNIT()
NAMED_UNIT(*)
SI_UNIT(.MILLI.,.METRE.)
);
#66724=(
NAMED_UNIT(*)
PLANE_ANGLE_UNIT()
SI_UNIT($,.RADIAN.)
);
#66725=(
NAMED_UNIT(*)
SI_UNIT($,.STERADIAN.)
SOLID_ANGLE_UNIT()
);
#66738=SHAPE_DEFINITION_REPRESENTATION(#66780,#66902);
#66780=PRODUCT_DEFINITION_SHAPE('',$,#66943);
#66902=SHAPE_REPRESENTATION('',(#27192),#66693);
#66930=PRODUCT_DEFINITION_CONTEXT('part definition',#67052,'design');
#66943=PRODUCT_DEFINITION('Slider End Cap','Slider End Cap',#66983,#66930);
#66983=PRODUCT_DEFINITION_FORMATION('',$,#67066);
#67052=APPLICATION_CONTEXT(
'Core Data for Automotive Mechanical Design Process');
#67053=PRODUCT_CONTEXT('part definition',#67052,'mechanical');
#67066=PRODUCT('Slider End Cap','Slider End Cap',$,(#67053));
#67095=PRESENTATION_STYLE_ASSIGNMENT((#67097));
#67097=SURFACE_STYLE_USAGE(.BOTH.,#67099);
#67099=SURFACE_SIDE_STYLE('',(#67101));
#67101=SURFACE_STYLE_FILL_AREA(#67103);
#67103=FILL_AREA_STYLE('Opaque(202,209,238)',(#67105));
#67105=FILL_AREA_STYLE_COLOUR('Opaque(202,209,238)',#67107);
#67107=COLOUR_RGB('Opaque(202,209,238)',0.792156862745098,0.819607843137255,
0.933333333333333);
ENDSEC;
END-ISO-10303-21;
